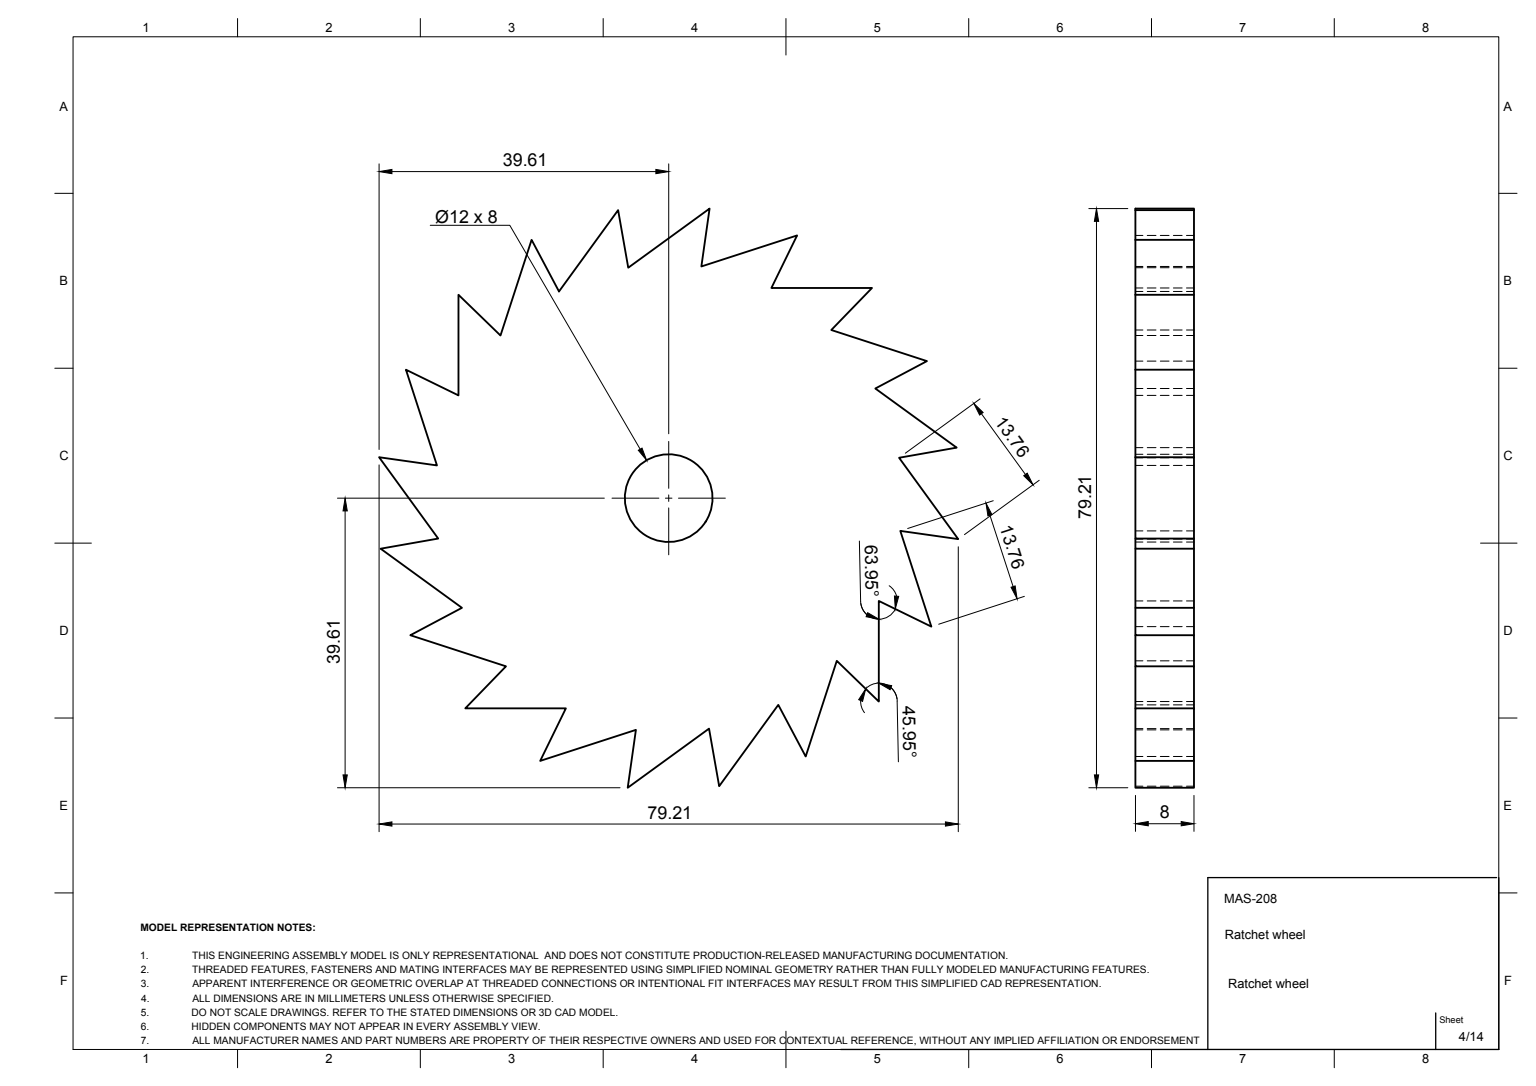
ISO-10303-21;
HEADER;
/* Generated by software containing ST-Developer
 * from STEP Tools, Inc. (www.steptools.com) 
 */

FILE_DESCRIPTION(
/* description */ ('Independent vertical20-tooth ratchet advance with repeated integral-c
ounterweight gravity pawls, swinging drive lever, bronze sleeves and f
ully retained axle stacks.18degpertooth. Native revolutes; geometric c
ycle checking rather than automatic contact/rolling dynamics. Gravity 
closing checked from actual pawl center of mass. Backplate/foot suppor
ts unit. Fits, torque, holding force, wear and life unassigned.'),
/* implementation_level */ '2;1');

FILE_NAME(
/* name */ 'Ratchet wheel.step',
/* time_stamp */ '2026-11-09T06:25:53-08:00',
/* author */ (''),
/* organization */ (''),
/* preprocessor_version */ 'ST-DEVELOPER v20.2',
/* originating_system */ 'Autodesk Translation Framework v15.17.0.0',
/* authorisation */ '');

FILE_SCHEMA (('AUTOMOTIVE_DESIGN { 1 0 10303 214 3 1 1 }'));
ENDSEC;

DATA;
#10=MECHANICAL_DESIGN_GEOMETRIC_PRESENTATION_REPRESENTATION('',(#124),#4643);
#96=SHAPE_REPRESENTATION_RELATIONSHIP('SRR','None',#4701,#110);
#110=ADVANCED_BREP_SHAPE_REPRESENTATION('',(#138),#4630);
#124=STYLED_ITEM('',(#4780),#138);
#138=MANIFOLD_SOLID_BREP('Body1',#2660);
#163=FACE_BOUND('',#523,.T.);
#164=FACE_BOUND('',#525,.T.);
#202=PLANE('',#2862);
#203=PLANE('',#2863);
#204=PLANE('',#2864);
#205=PLANE('',#2865);
#206=PLANE('',#2866);
#207=PLANE('',#2867);
#208=PLANE('',#2868);
#209=PLANE('',#2869);
#210=PLANE('',#2870);
#211=PLANE('',#2871);
#212=PLANE('',#2872);
#213=PLANE('',#2873);
#214=PLANE('',#2874);
#215=PLANE('',#2875);
#216=PLANE('',#2876);
#217=PLANE('',#2877);
#218=PLANE('',#2878);
#219=PLANE('',#2879);
#220=PLANE('',#2880);
#221=PLANE('',#2881);
#222=PLANE('',#2882);
#223=PLANE('',#2883);
#224=PLANE('',#2884);
#225=PLANE('',#2885);
#226=PLANE('',#2886);
#227=PLANE('',#2887);
#228=PLANE('',#2888);
#229=PLANE('',#2889);
#230=PLANE('',#2890);
#231=PLANE('',#2891);
#232=PLANE('',#2892);
#233=PLANE('',#2893);
#234=PLANE('',#2894);
#235=PLANE('',#2895);
#236=PLANE('',#2896);
#237=PLANE('',#2897);
#238=PLANE('',#2898);
#239=PLANE('',#2899);
#240=PLANE('',#2900);
#241=PLANE('',#2901);
#242=PLANE('',#2902);
#243=PLANE('',#2903);
#320=FACE_OUTER_BOUND('',#481,.T.);
#321=FACE_OUTER_BOUND('',#482,.T.);
#322=FACE_OUTER_BOUND('',#483,.T.);
#323=FACE_OUTER_BOUND('',#484,.T.);
#324=FACE_OUTER_BOUND('',#485,.T.);
#325=FACE_OUTER_BOUND('',#486,.T.);
#326=FACE_OUTER_BOUND('',#487,.T.);
#327=FACE_OUTER_BOUND('',#488,.T.);
#328=FACE_OUTER_BOUND('',#489,.T.);
#329=FACE_OUTER_BOUND('',#490,.T.);
#330=FACE_OUTER_BOUND('',#491,.T.);
#331=FACE_OUTER_BOUND('',#492,.T.);
#332=FACE_OUTER_BOUND('',#493,.T.);
#333=FACE_OUTER_BOUND('',#494,.T.);
#334=FACE_OUTER_BOUND('',#495,.T.);
#335=FACE_OUTER_BOUND('',#496,.T.);
#336=FACE_OUTER_BOUND('',#497,.T.);
#337=FACE_OUTER_BOUND('',#498,.T.);
#338=FACE_OUTER_BOUND('',#499,.T.);
#339=FACE_OUTER_BOUND('',#500,.T.);
#340=FACE_OUTER_BOUND('',#501,.T.);
#341=FACE_OUTER_BOUND('',#502,.T.);
#342=FACE_OUTER_BOUND('',#503,.T.);
#343=FACE_OUTER_BOUND('',#504,.T.);
#344=FACE_OUTER_BOUND('',#505,.T.);
#345=FACE_OUTER_BOUND('',#506,.T.);
#346=FACE_OUTER_BOUND('',#507,.T.);
#347=FACE_OUTER_BOUND('',#508,.T.);
#348=FACE_OUTER_BOUND('',#509,.T.);
#349=FACE_OUTER_BOUND('',#510,.T.);
#350=FACE_OUTER_BOUND('',#511,.T.);
#351=FACE_OUTER_BOUND('',#512,.T.);
#352=FACE_OUTER_BOUND('',#513,.T.);
#353=FACE_OUTER_BOUND('',#514,.T.);
#354=FACE_OUTER_BOUND('',#515,.T.);
#355=FACE_OUTER_BOUND('',#516,.T.);
#356=FACE_OUTER_BOUND('',#517,.T.);
#357=FACE_OUTER_BOUND('',#518,.T.);
#358=FACE_OUTER_BOUND('',#519,.T.);
#359=FACE_OUTER_BOUND('',#520,.T.);
#360=FACE_OUTER_BOUND('',#521,.T.);
#361=FACE_OUTER_BOUND('',#522,.T.);
#362=FACE_OUTER_BOUND('',#524,.T.);
#481=EDGE_LOOP('',(#1885,#1886,#1887,#1888));
#482=EDGE_LOOP('',(#1889,#1890,#1891,#1892));
#483=EDGE_LOOP('',(#1893,#1894,#1895,#1896));
#484=EDGE_LOOP('',(#1897,#1898,#1899,#1900));
#485=EDGE_LOOP('',(#1901,#1902,#1903,#1904));
#486=EDGE_LOOP('',(#1905,#1906,#1907,#1908));
#487=EDGE_LOOP('',(#1909,#1910,#1911,#1912));
#488=EDGE_LOOP('',(#1913,#1914,#1915,#1916));
#489=EDGE_LOOP('',(#1917,#1918,#1919,#1920));
#490=EDGE_LOOP('',(#1921,#1922,#1923,#1924));
#491=EDGE_LOOP('',(#1925,#1926,#1927,#1928));
#492=EDGE_LOOP('',(#1929,#1930,#1931,#1932));
#493=EDGE_LOOP('',(#1933,#1934,#1935,#1936));
#494=EDGE_LOOP('',(#1937,#1938,#1939,#1940));
#495=EDGE_LOOP('',(#1941,#1942,#1943,#1944));
#496=EDGE_LOOP('',(#1945,#1946,#1947,#1948));
#497=EDGE_LOOP('',(#1949,#1950,#1951,#1952));
#498=EDGE_LOOP('',(#1953,#1954,#1955,#1956));
#499=EDGE_LOOP('',(#1957,#1958,#1959,#1960));
#500=EDGE_LOOP('',(#1961,#1962,#1963,#1964));
#501=EDGE_LOOP('',(#1965,#1966,#1967,#1968));
#502=EDGE_LOOP('',(#1969,#1970,#1971,#1972));
#503=EDGE_LOOP('',(#1973,#1974,#1975,#1976));
#504=EDGE_LOOP('',(#1977,#1978,#1979,#1980));
#505=EDGE_LOOP('',(#1981,#1982,#1983,#1984));
#506=EDGE_LOOP('',(#1985,#1986,#1987,#1988));
#507=EDGE_LOOP('',(#1989,#1990,#1991,#1992));
#508=EDGE_LOOP('',(#1993,#1994,#1995,#1996));
#509=EDGE_LOOP('',(#1997,#1998,#1999,#2000));
#510=EDGE_LOOP('',(#2001,#2002,#2003,#2004));
#511=EDGE_LOOP('',(#2005,#2006,#2007,#2008));
#512=EDGE_LOOP('',(#2009,#2010,#2011,#2012));
#513=EDGE_LOOP('',(#2013,#2014,#2015,#2016));
#514=EDGE_LOOP('',(#2017,#2018,#2019,#2020));
#515=EDGE_LOOP('',(#2021,#2022,#2023,#2024));
#516=EDGE_LOOP('',(#2025,#2026,#2027,#2028));
#517=EDGE_LOOP('',(#2029,#2030,#2031,#2032));
#518=EDGE_LOOP('',(#2033,#2034,#2035,#2036));
#519=EDGE_LOOP('',(#2037,#2038,#2039,#2040));
#520=EDGE_LOOP('',(#2041,#2042,#2043,#2044));
#521=EDGE_LOOP('',(#2045,#2046,#2047,#2048));
#522=EDGE_LOOP('',(#2049,#2050,#2051,#2052,#2053,#2054,#2055,#2056,#2057,
#2058,#2059,#2060,#2061,#2062,#2063,#2064,#2065,#2066,#2067,#2068,#2069,
#2070,#2071,#2072,#2073,#2074,#2075,#2076,#2077,#2078,#2079,#2080,#2081,
#2082,#2083,#2084,#2085,#2086,#2087,#2088));
#523=EDGE_LOOP('',(#2089));
#524=EDGE_LOOP('',(#2090,#2091,#2092,#2093,#2094,#2095,#2096,#2097,#2098,
#2099,#2100,#2101,#2102,#2103,#2104,#2105,#2106,#2107,#2108,#2109,#2110,
#2111,#2112,#2113,#2114,#2115,#2116,#2117,#2118,#2119,#2120,#2121,#2122,
#2123,#2124,#2125,#2126,#2127,#2128,#2129));
#525=EDGE_LOOP('',(#2130));
#673=LINE('',#3960,#935);
#674=LINE('',#3965,#936);
#675=LINE('',#3967,#937);
#676=LINE('',#3969,#938);
#677=LINE('',#3970,#939);
#678=LINE('',#3973,#940);
#679=LINE('',#3975,#941);
#680=LINE('',#3976,#942);
#681=LINE('',#3979,#943);
#682=LINE('',#3981,#944);
#683=LINE('',#3982,#945);
#684=LINE('',#3985,#946);
#685=LINE('',#3987,#947);
#686=LINE('',#3988,#948);
#687=LINE('',#3991,#949);
#688=LINE('',#3993,#950);
#689=LINE('',#3994,#951);
#690=LINE('',#3997,#952);
#691=LINE('',#3999,#953);
#692=LINE('',#4000,#954);
#693=LINE('',#4003,#955);
#694=LINE('',#4005,#956);
#695=LINE('',#4006,#957);
#696=LINE('',#4009,#958);
#697=LINE('',#4011,#959);
#698=LINE('',#4012,#960);
#699=LINE('',#4015,#961);
#700=LINE('',#4017,#962);
#701=LINE('',#4018,#963);
#702=LINE('',#4021,#964);
#703=LINE('',#4023,#965);
#704=LINE('',#4024,#966);
#705=LINE('',#4027,#967);
#706=LINE('',#4029,#968);
#707=LINE('',#4030,#969);
#708=LINE('',#4033,#970);
#709=LINE('',#4035,#971);
#710=LINE('',#4036,#972);
#711=LINE('',#4039,#973);
#712=LINE('',#4041,#974);
#713=LINE('',#4042,#975);
#714=LINE('',#4045,#976);
#715=LINE('',#4047,#977);
#716=LINE('',#4048,#978);
#717=LINE('',#4051,#979);
#718=LINE('',#4053,#980);
#719=LINE('',#4054,#981);
#720=LINE('',#4057,#982);
#721=LINE('',#4059,#983);
#722=LINE('',#4060,#984);
#723=LINE('',#4063,#985);
#724=LINE('',#4065,#986);
#725=LINE('',#4066,#987);
#726=LINE('',#4069,#988);
#727=LINE('',#4071,#989);
#728=LINE('',#4072,#990);
#729=LINE('',#4075,#991);
#730=LINE('',#4077,#992);
#731=LINE('',#4078,#993);
#732=LINE('',#4081,#994);
#733=LINE('',#4083,#995);
#734=LINE('',#4084,#996);
#735=LINE('',#4087,#997);
#736=LINE('',#4089,#998);
#737=LINE('',#4090,#999);
#738=LINE('',#4093,#1000);
#739=LINE('',#4095,#1001);
#740=LINE('',#4096,#1002);
#741=LINE('',#4099,#1003);
#742=LINE('',#4101,#1004);
#743=LINE('',#4102,#1005);
#744=LINE('',#4105,#1006);
#745=LINE('',#4107,#1007);
#746=LINE('',#4108,#1008);
#747=LINE('',#4111,#1009);
#748=LINE('',#4113,#1010);
#749=LINE('',#4114,#1011);
#750=LINE('',#4117,#1012);
#751=LINE('',#4119,#1013);
#752=LINE('',#4120,#1014);
#753=LINE('',#4123,#1015);
#754=LINE('',#4125,#1016);
#755=LINE('',#4126,#1017);
#756=LINE('',#4129,#1018);
#757=LINE('',#4131,#1019);
#758=LINE('',#4132,#1020);
#759=LINE('',#4135,#1021);
#760=LINE('',#4137,#1022);
#761=LINE('',#4138,#1023);
#762=LINE('',#4141,#1024);
#763=LINE('',#4143,#1025);
#764=LINE('',#4144,#1026);
#765=LINE('',#4147,#1027);
#766=LINE('',#4149,#1028);
#767=LINE('',#4150,#1029);
#768=LINE('',#4153,#1030);
#769=LINE('',#4155,#1031);
#770=LINE('',#4156,#1032);
#771=LINE('',#4159,#1033);
#772=LINE('',#4161,#1034);
#773=LINE('',#4162,#1035);
#774=LINE('',#4165,#1036);
#775=LINE('',#4167,#1037);
#776=LINE('',#4168,#1038);
#777=LINE('',#4171,#1039);
#778=LINE('',#4173,#1040);
#779=LINE('',#4174,#1041);
#780=LINE('',#4177,#1042);
#781=LINE('',#4179,#1043);
#782=LINE('',#4180,#1044);
#783=LINE('',#4183,#1045);
#784=LINE('',#4185,#1046);
#785=LINE('',#4186,#1047);
#786=LINE('',#4189,#1048);
#787=LINE('',#4191,#1049);
#788=LINE('',#4192,#1050);
#789=LINE('',#4195,#1051);
#790=LINE('',#4197,#1052);
#791=LINE('',#4198,#1053);
#792=LINE('',#4200,#1054);
#793=LINE('',#4201,#1055);
#935=VECTOR('',#3183,6.);
#936=VECTOR('',#3188,10.);
#937=VECTOR('',#3189,10.);
#938=VECTOR('',#3190,10.);
#939=VECTOR('',#3191,10.);
#940=VECTOR('',#3194,10.);
#941=VECTOR('',#3195,10.);
#942=VECTOR('',#3196,10.);
#943=VECTOR('',#3199,10.);
#944=VECTOR('',#3200,10.);
#945=VECTOR('',#3201,10.);
#946=VECTOR('',#3204,10.);
#947=VECTOR('',#3205,10.);
#948=VECTOR('',#3206,10.);
#949=VECTOR('',#3209,10.);
#950=VECTOR('',#3210,10.);
#951=VECTOR('',#3211,10.);
#952=VECTOR('',#3214,10.);
#953=VECTOR('',#3215,10.);
#954=VECTOR('',#3216,10.);
#955=VECTOR('',#3219,10.);
#956=VECTOR('',#3220,10.);
#957=VECTOR('',#3221,10.);
#958=VECTOR('',#3224,10.);
#959=VECTOR('',#3225,10.);
#960=VECTOR('',#3226,10.);
#961=VECTOR('',#3229,10.);
#962=VECTOR('',#3230,10.);
#963=VECTOR('',#3231,10.);
#964=VECTOR('',#3234,10.);
#965=VECTOR('',#3235,10.);
#966=VECTOR('',#3236,10.);
#967=VECTOR('',#3239,10.);
#968=VECTOR('',#3240,10.);
#969=VECTOR('',#3241,10.);
#970=VECTOR('',#3244,10.);
#971=VECTOR('',#3245,10.);
#972=VECTOR('',#3246,10.);
#973=VECTOR('',#3249,10.);
#974=VECTOR('',#3250,10.);
#975=VECTOR('',#3251,10.);
#976=VECTOR('',#3254,10.);
#977=VECTOR('',#3255,10.);
#978=VECTOR('',#3256,10.);
#979=VECTOR('',#3259,10.);
#980=VECTOR('',#3260,10.);
#981=VECTOR('',#3261,10.);
#982=VECTOR('',#3264,10.);
#983=VECTOR('',#3265,10.);
#984=VECTOR('',#3266,10.);
#985=VECTOR('',#3269,10.);
#986=VECTOR('',#3270,10.);
#987=VECTOR('',#3271,10.);
#988=VECTOR('',#3274,10.);
#989=VECTOR('',#3275,10.);
#990=VECTOR('',#3276,10.);
#991=VECTOR('',#3279,10.);
#992=VECTOR('',#3280,10.);
#993=VECTOR('',#3281,10.);
#994=VECTOR('',#3284,10.);
#995=VECTOR('',#3285,10.);
#996=VECTOR('',#3286,10.);
#997=VECTOR('',#3289,10.);
#998=VECTOR('',#3290,10.);
#999=VECTOR('',#3291,10.);
#1000=VECTOR('',#3294,10.);
#1001=VECTOR('',#3295,10.);
#1002=VECTOR('',#3296,10.);
#1003=VECTOR('',#3299,10.);
#1004=VECTOR('',#3300,10.);
#1005=VECTOR('',#3301,10.);
#1006=VECTOR('',#3304,10.);
#1007=VECTOR('',#3305,10.);
#1008=VECTOR('',#3306,10.);
#1009=VECTOR('',#3309,10.);
#1010=VECTOR('',#3310,10.);
#1011=VECTOR('',#3311,10.);
#1012=VECTOR('',#3314,10.);
#1013=VECTOR('',#3315,10.);
#1014=VECTOR('',#3316,10.);
#1015=VECTOR('',#3319,10.);
#1016=VECTOR('',#3320,10.);
#1017=VECTOR('',#3321,10.);
#1018=VECTOR('',#3324,10.);
#1019=VECTOR('',#3325,10.);
#1020=VECTOR('',#3326,10.);
#1021=VECTOR('',#3329,10.);
#1022=VECTOR('',#3330,10.);
#1023=VECTOR('',#3331,10.);
#1024=VECTOR('',#3334,10.);
#1025=VECTOR('',#3335,10.);
#1026=VECTOR('',#3336,10.);
#1027=VECTOR('',#3339,10.);
#1028=VECTOR('',#3340,10.);
#1029=VECTOR('',#3341,10.);
#1030=VECTOR('',#3344,10.);
#1031=VECTOR('',#3345,10.);
#1032=VECTOR('',#3346,10.);
#1033=VECTOR('',#3349,10.);
#1034=VECTOR('',#3350,10.);
#1035=VECTOR('',#3351,10.);
#1036=VECTOR('',#3354,10.);
#1037=VECTOR('',#3355,10.);
#1038=VECTOR('',#3356,10.);
#1039=VECTOR('',#3359,10.);
#1040=VECTOR('',#3360,10.);
#1041=VECTOR('',#3361,10.);
#1042=VECTOR('',#3364,10.);
#1043=VECTOR('',#3365,10.);
#1044=VECTOR('',#3366,10.);
#1045=VECTOR('',#3369,10.);
#1046=VECTOR('',#3370,10.);
#1047=VECTOR('',#3371,10.);
#1048=VECTOR('',#3374,10.);
#1049=VECTOR('',#3375,10.);
#1050=VECTOR('',#3376,10.);
#1051=VECTOR('',#3379,10.);
#1052=VECTOR('',#3380,10.);
#1053=VECTOR('',#3381,10.);
#1054=VECTOR('',#3384,10.);
#1055=VECTOR('',#3385,10.);
#1179=CIRCLE('',#2860,6.);
#1180=CIRCLE('',#2861,6.);
#1269=VERTEX_POINT('',#3957);
#1270=VERTEX_POINT('',#3959);
#1271=VERTEX_POINT('',#3963);
#1272=VERTEX_POINT('',#3964);
#1273=VERTEX_POINT('',#3966);
#1274=VERTEX_POINT('',#3968);
#1275=VERTEX_POINT('',#3972);
#1276=VERTEX_POINT('',#3974);
#1277=VERTEX_POINT('',#3978);
#1278=VERTEX_POINT('',#3980);
#1279=VERTEX_POINT('',#3984);
#1280=VERTEX_POINT('',#3986);
#1281=VERTEX_POINT('',#3990);
#1282=VERTEX_POINT('',#3992);
#1283=VERTEX_POINT('',#3996);
#1284=VERTEX_POINT('',#3998);
#1285=VERTEX_POINT('',#4002);
#1286=VERTEX_POINT('',#4004);
#1287=VERTEX_POINT('',#4008);
#1288=VERTEX_POINT('',#4010);
#1289=VERTEX_POINT('',#4014);
#1290=VERTEX_POINT('',#4016);
#1291=VERTEX_POINT('',#4020);
#1292=VERTEX_POINT('',#4022);
#1293=VERTEX_POINT('',#4026);
#1294=VERTEX_POINT('',#4028);
#1295=VERTEX_POINT('',#4032);
#1296=VERTEX_POINT('',#4034);
#1297=VERTEX_POINT('',#4038);
#1298=VERTEX_POINT('',#4040);
#1299=VERTEX_POINT('',#4044);
#1300=VERTEX_POINT('',#4046);
#1301=VERTEX_POINT('',#4050);
#1302=VERTEX_POINT('',#4052);
#1303=VERTEX_POINT('',#4056);
#1304=VERTEX_POINT('',#4058);
#1305=VERTEX_POINT('',#4062);
#1306=VERTEX_POINT('',#4064);
#1307=VERTEX_POINT('',#4068);
#1308=VERTEX_POINT('',#4070);
#1309=VERTEX_POINT('',#4074);
#1310=VERTEX_POINT('',#4076);
#1311=VERTEX_POINT('',#4080);
#1312=VERTEX_POINT('',#4082);
#1313=VERTEX_POINT('',#4086);
#1314=VERTEX_POINT('',#4088);
#1315=VERTEX_POINT('',#4092);
#1316=VERTEX_POINT('',#4094);
#1317=VERTEX_POINT('',#4098);
#1318=VERTEX_POINT('',#4100);
#1319=VERTEX_POINT('',#4104);
#1320=VERTEX_POINT('',#4106);
#1321=VERTEX_POINT('',#4110);
#1322=VERTEX_POINT('',#4112);
#1323=VERTEX_POINT('',#4116);
#1324=VERTEX_POINT('',#4118);
#1325=VERTEX_POINT('',#4122);
#1326=VERTEX_POINT('',#4124);
#1327=VERTEX_POINT('',#4128);
#1328=VERTEX_POINT('',#4130);
#1329=VERTEX_POINT('',#4134);
#1330=VERTEX_POINT('',#4136);
#1331=VERTEX_POINT('',#4140);
#1332=VERTEX_POINT('',#4142);
#1333=VERTEX_POINT('',#4146);
#1334=VERTEX_POINT('',#4148);
#1335=VERTEX_POINT('',#4152);
#1336=VERTEX_POINT('',#4154);
#1337=VERTEX_POINT('',#4158);
#1338=VERTEX_POINT('',#4160);
#1339=VERTEX_POINT('',#4164);
#1340=VERTEX_POINT('',#4166);
#1341=VERTEX_POINT('',#4170);
#1342=VERTEX_POINT('',#4172);
#1343=VERTEX_POINT('',#4176);
#1344=VERTEX_POINT('',#4178);
#1345=VERTEX_POINT('',#4182);
#1346=VERTEX_POINT('',#4184);
#1347=VERTEX_POINT('',#4188);
#1348=VERTEX_POINT('',#4190);
#1349=VERTEX_POINT('',#4194);
#1350=VERTEX_POINT('',#4196);
#1507=EDGE_CURVE('',#1269,#1269,#1179,.T.);
#1508=EDGE_CURVE('',#1269,#1270,#673,.T.);
#1509=EDGE_CURVE('',#1270,#1270,#1180,.T.);
#1510=EDGE_CURVE('',#1271,#1272,#674,.T.);
#1511=EDGE_CURVE('',#1272,#1273,#675,.T.);
#1512=EDGE_CURVE('',#1274,#1273,#676,.T.);
#1513=EDGE_CURVE('',#1271,#1274,#677,.T.);
#1514=EDGE_CURVE('',#1275,#1271,#678,.T.);
#1515=EDGE_CURVE('',#1276,#1274,#679,.T.);
#1516=EDGE_CURVE('',#1275,#1276,#680,.T.);
#1517=EDGE_CURVE('',#1277,#1275,#681,.T.);
#1518=EDGE_CURVE('',#1278,#1276,#682,.T.);
#1519=EDGE_CURVE('',#1277,#1278,#683,.T.);
#1520=EDGE_CURVE('',#1279,#1277,#684,.T.);
#1521=EDGE_CURVE('',#1280,#1278,#685,.T.);
#1522=EDGE_CURVE('',#1279,#1280,#686,.T.);
#1523=EDGE_CURVE('',#1281,#1279,#687,.T.);
#1524=EDGE_CURVE('',#1282,#1280,#688,.T.);
#1525=EDGE_CURVE('',#1281,#1282,#689,.T.);
#1526=EDGE_CURVE('',#1283,#1281,#690,.T.);
#1527=EDGE_CURVE('',#1284,#1282,#691,.T.);
#1528=EDGE_CURVE('',#1283,#1284,#692,.T.);
#1529=EDGE_CURVE('',#1285,#1283,#693,.T.);
#1530=EDGE_CURVE('',#1286,#1284,#694,.T.);
#1531=EDGE_CURVE('',#1285,#1286,#695,.T.);
#1532=EDGE_CURVE('',#1287,#1285,#696,.T.);
#1533=EDGE_CURVE('',#1288,#1286,#697,.T.);
#1534=EDGE_CURVE('',#1287,#1288,#698,.T.);
#1535=EDGE_CURVE('',#1289,#1287,#699,.T.);
#1536=EDGE_CURVE('',#1290,#1288,#700,.T.);
#1537=EDGE_CURVE('',#1289,#1290,#701,.T.);
#1538=EDGE_CURVE('',#1291,#1289,#702,.T.);
#1539=EDGE_CURVE('',#1292,#1290,#703,.T.);
#1540=EDGE_CURVE('',#1291,#1292,#704,.T.);
#1541=EDGE_CURVE('',#1293,#1291,#705,.T.);
#1542=EDGE_CURVE('',#1294,#1292,#706,.T.);
#1543=EDGE_CURVE('',#1293,#1294,#707,.T.);
#1544=EDGE_CURVE('',#1295,#1293,#708,.T.);
#1545=EDGE_CURVE('',#1296,#1294,#709,.T.);
#1546=EDGE_CURVE('',#1295,#1296,#710,.T.);
#1547=EDGE_CURVE('',#1297,#1295,#711,.T.);
#1548=EDGE_CURVE('',#1298,#1296,#712,.T.);
#1549=EDGE_CURVE('',#1297,#1298,#713,.T.);
#1550=EDGE_CURVE('',#1299,#1297,#714,.T.);
#1551=EDGE_CURVE('',#1300,#1298,#715,.T.);
#1552=EDGE_CURVE('',#1299,#1300,#716,.T.);
#1553=EDGE_CURVE('',#1301,#1299,#717,.T.);
#1554=EDGE_CURVE('',#1302,#1300,#718,.T.);
#1555=EDGE_CURVE('',#1301,#1302,#719,.T.);
#1556=EDGE_CURVE('',#1303,#1301,#720,.T.);
#1557=EDGE_CURVE('',#1304,#1302,#721,.T.);
#1558=EDGE_CURVE('',#1303,#1304,#722,.T.);
#1559=EDGE_CURVE('',#1305,#1303,#723,.T.);
#1560=EDGE_CURVE('',#1306,#1304,#724,.T.);
#1561=EDGE_CURVE('',#1305,#1306,#725,.T.);
#1562=EDGE_CURVE('',#1307,#1305,#726,.T.);
#1563=EDGE_CURVE('',#1308,#1306,#727,.T.);
#1564=EDGE_CURVE('',#1307,#1308,#728,.T.);
#1565=EDGE_CURVE('',#1309,#1307,#729,.T.);
#1566=EDGE_CURVE('',#1310,#1308,#730,.T.);
#1567=EDGE_CURVE('',#1309,#1310,#731,.T.);
#1568=EDGE_CURVE('',#1311,#1309,#732,.T.);
#1569=EDGE_CURVE('',#1312,#1310,#733,.T.);
#1570=EDGE_CURVE('',#1311,#1312,#734,.T.);
#1571=EDGE_CURVE('',#1313,#1311,#735,.T.);
#1572=EDGE_CURVE('',#1314,#1312,#736,.T.);
#1573=EDGE_CURVE('',#1313,#1314,#737,.T.);
#1574=EDGE_CURVE('',#1315,#1313,#738,.T.);
#1575=EDGE_CURVE('',#1316,#1314,#739,.T.);
#1576=EDGE_CURVE('',#1315,#1316,#740,.T.);
#1577=EDGE_CURVE('',#1317,#1315,#741,.T.);
#1578=EDGE_CURVE('',#1318,#1316,#742,.T.);
#1579=EDGE_CURVE('',#1317,#1318,#743,.T.);
#1580=EDGE_CURVE('',#1319,#1317,#744,.T.);
#1581=EDGE_CURVE('',#1320,#1318,#745,.T.);
#1582=EDGE_CURVE('',#1319,#1320,#746,.T.);
#1583=EDGE_CURVE('',#1321,#1319,#747,.T.);
#1584=EDGE_CURVE('',#1322,#1320,#748,.T.);
#1585=EDGE_CURVE('',#1321,#1322,#749,.T.);
#1586=EDGE_CURVE('',#1323,#1321,#750,.T.);
#1587=EDGE_CURVE('',#1324,#1322,#751,.T.);
#1588=EDGE_CURVE('',#1323,#1324,#752,.T.);
#1589=EDGE_CURVE('',#1325,#1323,#753,.T.);
#1590=EDGE_CURVE('',#1326,#1324,#754,.T.);
#1591=EDGE_CURVE('',#1325,#1326,#755,.T.);
#1592=EDGE_CURVE('',#1327,#1325,#756,.T.);
#1593=EDGE_CURVE('',#1328,#1326,#757,.T.);
#1594=EDGE_CURVE('',#1327,#1328,#758,.T.);
#1595=EDGE_CURVE('',#1329,#1327,#759,.T.);
#1596=EDGE_CURVE('',#1330,#1328,#760,.T.);
#1597=EDGE_CURVE('',#1329,#1330,#761,.T.);
#1598=EDGE_CURVE('',#1331,#1329,#762,.T.);
#1599=EDGE_CURVE('',#1332,#1330,#763,.T.);
#1600=EDGE_CURVE('',#1331,#1332,#764,.T.);
#1601=EDGE_CURVE('',#1333,#1331,#765,.T.);
#1602=EDGE_CURVE('',#1334,#1332,#766,.T.);
#1603=EDGE_CURVE('',#1333,#1334,#767,.T.);
#1604=EDGE_CURVE('',#1335,#1333,#768,.T.);
#1605=EDGE_CURVE('',#1336,#1334,#769,.T.);
#1606=EDGE_CURVE('',#1335,#1336,#770,.T.);
#1607=EDGE_CURVE('',#1337,#1335,#771,.T.);
#1608=EDGE_CURVE('',#1338,#1336,#772,.T.);
#1609=EDGE_CURVE('',#1337,#1338,#773,.T.);
#1610=EDGE_CURVE('',#1339,#1337,#774,.T.);
#1611=EDGE_CURVE('',#1340,#1338,#775,.T.);
#1612=EDGE_CURVE('',#1339,#1340,#776,.T.);
#1613=EDGE_CURVE('',#1341,#1339,#777,.T.);
#1614=EDGE_CURVE('',#1342,#1340,#778,.T.);
#1615=EDGE_CURVE('',#1341,#1342,#779,.T.);
#1616=EDGE_CURVE('',#1343,#1341,#780,.T.);
#1617=EDGE_CURVE('',#1344,#1342,#781,.T.);
#1618=EDGE_CURVE('',#1343,#1344,#782,.T.);
#1619=EDGE_CURVE('',#1345,#1343,#783,.T.);
#1620=EDGE_CURVE('',#1346,#1344,#784,.T.);
#1621=EDGE_CURVE('',#1345,#1346,#785,.T.);
#1622=EDGE_CURVE('',#1347,#1345,#786,.T.);
#1623=EDGE_CURVE('',#1348,#1346,#787,.T.);
#1624=EDGE_CURVE('',#1347,#1348,#788,.T.);
#1625=EDGE_CURVE('',#1349,#1347,#789,.T.);
#1626=EDGE_CURVE('',#1350,#1348,#790,.T.);
#1627=EDGE_CURVE('',#1349,#1350,#791,.T.);
#1628=EDGE_CURVE('',#1272,#1349,#792,.T.);
#1629=EDGE_CURVE('',#1273,#1350,#793,.T.);
#1885=ORIENTED_EDGE('',*,*,#1507,.F.);
#1886=ORIENTED_EDGE('',*,*,#1508,.T.);
#1887=ORIENTED_EDGE('',*,*,#1509,.F.);
#1888=ORIENTED_EDGE('',*,*,#1508,.F.);
#1889=ORIENTED_EDGE('',*,*,#1510,.T.);
#1890=ORIENTED_EDGE('',*,*,#1511,.T.);
#1891=ORIENTED_EDGE('',*,*,#1512,.F.);
#1892=ORIENTED_EDGE('',*,*,#1513,.F.);
#1893=ORIENTED_EDGE('',*,*,#1514,.T.);
#1894=ORIENTED_EDGE('',*,*,#1513,.T.);
#1895=ORIENTED_EDGE('',*,*,#1515,.F.);
#1896=ORIENTED_EDGE('',*,*,#1516,.F.);
#1897=ORIENTED_EDGE('',*,*,#1517,.T.);
#1898=ORIENTED_EDGE('',*,*,#1516,.T.);
#1899=ORIENTED_EDGE('',*,*,#1518,.F.);
#1900=ORIENTED_EDGE('',*,*,#1519,.F.);
#1901=ORIENTED_EDGE('',*,*,#1520,.T.);
#1902=ORIENTED_EDGE('',*,*,#1519,.T.);
#1903=ORIENTED_EDGE('',*,*,#1521,.F.);
#1904=ORIENTED_EDGE('',*,*,#1522,.F.);
#1905=ORIENTED_EDGE('',*,*,#1523,.T.);
#1906=ORIENTED_EDGE('',*,*,#1522,.T.);
#1907=ORIENTED_EDGE('',*,*,#1524,.F.);
#1908=ORIENTED_EDGE('',*,*,#1525,.F.);
#1909=ORIENTED_EDGE('',*,*,#1526,.T.);
#1910=ORIENTED_EDGE('',*,*,#1525,.T.);
#1911=ORIENTED_EDGE('',*,*,#1527,.F.);
#1912=ORIENTED_EDGE('',*,*,#1528,.F.);
#1913=ORIENTED_EDGE('',*,*,#1529,.T.);
#1914=ORIENTED_EDGE('',*,*,#1528,.T.);
#1915=ORIENTED_EDGE('',*,*,#1530,.F.);
#1916=ORIENTED_EDGE('',*,*,#1531,.F.);
#1917=ORIENTED_EDGE('',*,*,#1532,.T.);
#1918=ORIENTED_EDGE('',*,*,#1531,.T.);
#1919=ORIENTED_EDGE('',*,*,#1533,.F.);
#1920=ORIENTED_EDGE('',*,*,#1534,.F.);
#1921=ORIENTED_EDGE('',*,*,#1535,.T.);
#1922=ORIENTED_EDGE('',*,*,#1534,.T.);
#1923=ORIENTED_EDGE('',*,*,#1536,.F.);
#1924=ORIENTED_EDGE('',*,*,#1537,.F.);
#1925=ORIENTED_EDGE('',*,*,#1538,.T.);
#1926=ORIENTED_EDGE('',*,*,#1537,.T.);
#1927=ORIENTED_EDGE('',*,*,#1539,.F.);
#1928=ORIENTED_EDGE('',*,*,#1540,.F.);
#1929=ORIENTED_EDGE('',*,*,#1541,.T.);
#1930=ORIENTED_EDGE('',*,*,#1540,.T.);
#1931=ORIENTED_EDGE('',*,*,#1542,.F.);
#1932=ORIENTED_EDGE('',*,*,#1543,.F.);
#1933=ORIENTED_EDGE('',*,*,#1544,.T.);
#1934=ORIENTED_EDGE('',*,*,#1543,.T.);
#1935=ORIENTED_EDGE('',*,*,#1545,.F.);
#1936=ORIENTED_EDGE('',*,*,#1546,.F.);
#1937=ORIENTED_EDGE('',*,*,#1547,.T.);
#1938=ORIENTED_EDGE('',*,*,#1546,.T.);
#1939=ORIENTED_EDGE('',*,*,#1548,.F.);
#1940=ORIENTED_EDGE('',*,*,#1549,.F.);
#1941=ORIENTED_EDGE('',*,*,#1550,.T.);
#1942=ORIENTED_EDGE('',*,*,#1549,.T.);
#1943=ORIENTED_EDGE('',*,*,#1551,.F.);
#1944=ORIENTED_EDGE('',*,*,#1552,.F.);
#1945=ORIENTED_EDGE('',*,*,#1553,.T.);
#1946=ORIENTED_EDGE('',*,*,#1552,.T.);
#1947=ORIENTED_EDGE('',*,*,#1554,.F.);
#1948=ORIENTED_EDGE('',*,*,#1555,.F.);
#1949=ORIENTED_EDGE('',*,*,#1556,.T.);
#1950=ORIENTED_EDGE('',*,*,#1555,.T.);
#1951=ORIENTED_EDGE('',*,*,#1557,.F.);
#1952=ORIENTED_EDGE('',*,*,#1558,.F.);
#1953=ORIENTED_EDGE('',*,*,#1559,.T.);
#1954=ORIENTED_EDGE('',*,*,#1558,.T.);
#1955=ORIENTED_EDGE('',*,*,#1560,.F.);
#1956=ORIENTED_EDGE('',*,*,#1561,.F.);
#1957=ORIENTED_EDGE('',*,*,#1562,.T.);
#1958=ORIENTED_EDGE('',*,*,#1561,.T.);
#1959=ORIENTED_EDGE('',*,*,#1563,.F.);
#1960=ORIENTED_EDGE('',*,*,#1564,.F.);
#1961=ORIENTED_EDGE('',*,*,#1565,.T.);
#1962=ORIENTED_EDGE('',*,*,#1564,.T.);
#1963=ORIENTED_EDGE('',*,*,#1566,.F.);
#1964=ORIENTED_EDGE('',*,*,#1567,.F.);
#1965=ORIENTED_EDGE('',*,*,#1568,.T.);
#1966=ORIENTED_EDGE('',*,*,#1567,.T.);
#1967=ORIENTED_EDGE('',*,*,#1569,.F.);
#1968=ORIENTED_EDGE('',*,*,#1570,.F.);
#1969=ORIENTED_EDGE('',*,*,#1571,.T.);
#1970=ORIENTED_EDGE('',*,*,#1570,.T.);
#1971=ORIENTED_EDGE('',*,*,#1572,.F.);
#1972=ORIENTED_EDGE('',*,*,#1573,.F.);
#1973=ORIENTED_EDGE('',*,*,#1574,.T.);
#1974=ORIENTED_EDGE('',*,*,#1573,.T.);
#1975=ORIENTED_EDGE('',*,*,#1575,.F.);
#1976=ORIENTED_EDGE('',*,*,#1576,.F.);
#1977=ORIENTED_EDGE('',*,*,#1577,.T.);
#1978=ORIENTED_EDGE('',*,*,#1576,.T.);
#1979=ORIENTED_EDGE('',*,*,#1578,.F.);
#1980=ORIENTED_EDGE('',*,*,#1579,.F.);
#1981=ORIENTED_EDGE('',*,*,#1580,.T.);
#1982=ORIENTED_EDGE('',*,*,#1579,.T.);
#1983=ORIENTED_EDGE('',*,*,#1581,.F.);
#1984=ORIENTED_EDGE('',*,*,#1582,.F.);
#1985=ORIENTED_EDGE('',*,*,#1583,.T.);
#1986=ORIENTED_EDGE('',*,*,#1582,.T.);
#1987=ORIENTED_EDGE('',*,*,#1584,.F.);
#1988=ORIENTED_EDGE('',*,*,#1585,.F.);
#1989=ORIENTED_EDGE('',*,*,#1586,.T.);
#1990=ORIENTED_EDGE('',*,*,#1585,.T.);
#1991=ORIENTED_EDGE('',*,*,#1587,.F.);
#1992=ORIENTED_EDGE('',*,*,#1588,.F.);
#1993=ORIENTED_EDGE('',*,*,#1589,.T.);
#1994=ORIENTED_EDGE('',*,*,#1588,.T.);
#1995=ORIENTED_EDGE('',*,*,#1590,.F.);
#1996=ORIENTED_EDGE('',*,*,#1591,.F.);
#1997=ORIENTED_EDGE('',*,*,#1592,.T.);
#1998=ORIENTED_EDGE('',*,*,#1591,.T.);
#1999=ORIENTED_EDGE('',*,*,#1593,.F.);
#2000=ORIENTED_EDGE('',*,*,#1594,.F.);
#2001=ORIENTED_EDGE('',*,*,#1595,.T.);
#2002=ORIENTED_EDGE('',*,*,#1594,.T.);
#2003=ORIENTED_EDGE('',*,*,#1596,.F.);
#2004=ORIENTED_EDGE('',*,*,#1597,.F.);
#2005=ORIENTED_EDGE('',*,*,#1598,.T.);
#2006=ORIENTED_EDGE('',*,*,#1597,.T.);
#2007=ORIENTED_EDGE('',*,*,#1599,.F.);
#2008=ORIENTED_EDGE('',*,*,#1600,.F.);
#2009=ORIENTED_EDGE('',*,*,#1601,.T.);
#2010=ORIENTED_EDGE('',*,*,#1600,.T.);
#2011=ORIENTED_EDGE('',*,*,#1602,.F.);
#2012=ORIENTED_EDGE('',*,*,#1603,.F.);
#2013=ORIENTED_EDGE('',*,*,#1604,.T.);
#2014=ORIENTED_EDGE('',*,*,#1603,.T.);
#2015=ORIENTED_EDGE('',*,*,#1605,.F.);
#2016=ORIENTED_EDGE('',*,*,#1606,.F.);
#2017=ORIENTED_EDGE('',*,*,#1607,.T.);
#2018=ORIENTED_EDGE('',*,*,#1606,.T.);
#2019=ORIENTED_EDGE('',*,*,#1608,.F.);
#2020=ORIENTED_EDGE('',*,*,#1609,.F.);
#2021=ORIENTED_EDGE('',*,*,#1610,.T.);
#2022=ORIENTED_EDGE('',*,*,#1609,.T.);
#2023=ORIENTED_EDGE('',*,*,#1611,.F.);
#2024=ORIENTED_EDGE('',*,*,#1612,.F.);
#2025=ORIENTED_EDGE('',*,*,#1613,.T.);
#2026=ORIENTED_EDGE('',*,*,#1612,.T.);
#2027=ORIENTED_EDGE('',*,*,#1614,.F.);
#2028=ORIENTED_EDGE('',*,*,#1615,.F.);
#2029=ORIENTED_EDGE('',*,*,#1616,.T.);
#2030=ORIENTED_EDGE('',*,*,#1615,.T.);
#2031=ORIENTED_EDGE('',*,*,#1617,.F.);
#2032=ORIENTED_EDGE('',*,*,#1618,.F.);
#2033=ORIENTED_EDGE('',*,*,#1619,.T.);
#2034=ORIENTED_EDGE('',*,*,#1618,.T.);
#2035=ORIENTED_EDGE('',*,*,#1620,.F.);
#2036=ORIENTED_EDGE('',*,*,#1621,.F.);
#2037=ORIENTED_EDGE('',*,*,#1622,.T.);
#2038=ORIENTED_EDGE('',*,*,#1621,.T.);
#2039=ORIENTED_EDGE('',*,*,#1623,.F.);
#2040=ORIENTED_EDGE('',*,*,#1624,.F.);
#2041=ORIENTED_EDGE('',*,*,#1625,.T.);
#2042=ORIENTED_EDGE('',*,*,#1624,.T.);
#2043=ORIENTED_EDGE('',*,*,#1626,.F.);
#2044=ORIENTED_EDGE('',*,*,#1627,.F.);
#2045=ORIENTED_EDGE('',*,*,#1628,.T.);
#2046=ORIENTED_EDGE('',*,*,#1627,.T.);
#2047=ORIENTED_EDGE('',*,*,#1629,.F.);
#2048=ORIENTED_EDGE('',*,*,#1511,.F.);
#2049=ORIENTED_EDGE('',*,*,#1629,.T.);
#2050=ORIENTED_EDGE('',*,*,#1626,.T.);
#2051=ORIENTED_EDGE('',*,*,#1623,.T.);
#2052=ORIENTED_EDGE('',*,*,#1620,.T.);
#2053=ORIENTED_EDGE('',*,*,#1617,.T.);
#2054=ORIENTED_EDGE('',*,*,#1614,.T.);
#2055=ORIENTED_EDGE('',*,*,#1611,.T.);
#2056=ORIENTED_EDGE('',*,*,#1608,.T.);
#2057=ORIENTED_EDGE('',*,*,#1605,.T.);
#2058=ORIENTED_EDGE('',*,*,#1602,.T.);
#2059=ORIENTED_EDGE('',*,*,#1599,.T.);
#2060=ORIENTED_EDGE('',*,*,#1596,.T.);
#2061=ORIENTED_EDGE('',*,*,#1593,.T.);
#2062=ORIENTED_EDGE('',*,*,#1590,.T.);
#2063=ORIENTED_EDGE('',*,*,#1587,.T.);
#2064=ORIENTED_EDGE('',*,*,#1584,.T.);
#2065=ORIENTED_EDGE('',*,*,#1581,.T.);
#2066=ORIENTED_EDGE('',*,*,#1578,.T.);
#2067=ORIENTED_EDGE('',*,*,#1575,.T.);
#2068=ORIENTED_EDGE('',*,*,#1572,.T.);
#2069=ORIENTED_EDGE('',*,*,#1569,.T.);
#2070=ORIENTED_EDGE('',*,*,#1566,.T.);
#2071=ORIENTED_EDGE('',*,*,#1563,.T.);
#2072=ORIENTED_EDGE('',*,*,#1560,.T.);
#2073=ORIENTED_EDGE('',*,*,#1557,.T.);
#2074=ORIENTED_EDGE('',*,*,#1554,.T.);
#2075=ORIENTED_EDGE('',*,*,#1551,.T.);
#2076=ORIENTED_EDGE('',*,*,#1548,.T.);
#2077=ORIENTED_EDGE('',*,*,#1545,.T.);
#2078=ORIENTED_EDGE('',*,*,#1542,.T.);
#2079=ORIENTED_EDGE('',*,*,#1539,.T.);
#2080=ORIENTED_EDGE('',*,*,#1536,.T.);
#2081=ORIENTED_EDGE('',*,*,#1533,.T.);
#2082=ORIENTED_EDGE('',*,*,#1530,.T.);
#2083=ORIENTED_EDGE('',*,*,#1527,.T.);
#2084=ORIENTED_EDGE('',*,*,#1524,.T.);
#2085=ORIENTED_EDGE('',*,*,#1521,.T.);
#2086=ORIENTED_EDGE('',*,*,#1518,.T.);
#2087=ORIENTED_EDGE('',*,*,#1515,.T.);
#2088=ORIENTED_EDGE('',*,*,#1512,.T.);
#2089=ORIENTED_EDGE('',*,*,#1507,.T.);
#2090=ORIENTED_EDGE('',*,*,#1628,.F.);
#2091=ORIENTED_EDGE('',*,*,#1510,.F.);
#2092=ORIENTED_EDGE('',*,*,#1514,.F.);
#2093=ORIENTED_EDGE('',*,*,#1517,.F.);
#2094=ORIENTED_EDGE('',*,*,#1520,.F.);
#2095=ORIENTED_EDGE('',*,*,#1523,.F.);
#2096=ORIENTED_EDGE('',*,*,#1526,.F.);
#2097=ORIENTED_EDGE('',*,*,#1529,.F.);
#2098=ORIENTED_EDGE('',*,*,#1532,.F.);
#2099=ORIENTED_EDGE('',*,*,#1535,.F.);
#2100=ORIENTED_EDGE('',*,*,#1538,.F.);
#2101=ORIENTED_EDGE('',*,*,#1541,.F.);
#2102=ORIENTED_EDGE('',*,*,#1544,.F.);
#2103=ORIENTED_EDGE('',*,*,#1547,.F.);
#2104=ORIENTED_EDGE('',*,*,#1550,.F.);
#2105=ORIENTED_EDGE('',*,*,#1553,.F.);
#2106=ORIENTED_EDGE('',*,*,#1556,.F.);
#2107=ORIENTED_EDGE('',*,*,#1559,.F.);
#2108=ORIENTED_EDGE('',*,*,#1562,.F.);
#2109=ORIENTED_EDGE('',*,*,#1565,.F.);
#2110=ORIENTED_EDGE('',*,*,#1568,.F.);
#2111=ORIENTED_EDGE('',*,*,#1571,.F.);
#2112=ORIENTED_EDGE('',*,*,#1574,.F.);
#2113=ORIENTED_EDGE('',*,*,#1577,.F.);
#2114=ORIENTED_EDGE('',*,*,#1580,.F.);
#2115=ORIENTED_EDGE('',*,*,#1583,.F.);
#2116=ORIENTED_EDGE('',*,*,#1586,.F.);
#2117=ORIENTED_EDGE('',*,*,#1589,.F.);
#2118=ORIENTED_EDGE('',*,*,#1592,.F.);
#2119=ORIENTED_EDGE('',*,*,#1595,.F.);
#2120=ORIENTED_EDGE('',*,*,#1598,.F.);
#2121=ORIENTED_EDGE('',*,*,#1601,.F.);
#2122=ORIENTED_EDGE('',*,*,#1604,.F.);
#2123=ORIENTED_EDGE('',*,*,#1607,.F.);
#2124=ORIENTED_EDGE('',*,*,#1610,.F.);
#2125=ORIENTED_EDGE('',*,*,#1613,.F.);
#2126=ORIENTED_EDGE('',*,*,#1616,.F.);
#2127=ORIENTED_EDGE('',*,*,#1619,.F.);
#2128=ORIENTED_EDGE('',*,*,#1622,.F.);
#2129=ORIENTED_EDGE('',*,*,#1625,.F.);
#2130=ORIENTED_EDGE('',*,*,#1509,.T.);
#2479=CYLINDRICAL_SURFACE('',#2859,6.);
#2526=ADVANCED_FACE('',(#320),#2479,.F.);
#2527=ADVANCED_FACE('',(#321),#202,.T.);
#2528=ADVANCED_FACE('',(#322),#203,.T.);
#2529=ADVANCED_FACE('',(#323),#204,.T.);
#2530=ADVANCED_FACE('',(#324),#205,.T.);
#2531=ADVANCED_FACE('',(#325),#206,.T.);
#2532=ADVANCED_FACE('',(#326),#207,.T.);
#2533=ADVANCED_FACE('',(#327),#208,.T.);
#2534=ADVANCED_FACE('',(#328),#209,.T.);
#2535=ADVANCED_FACE('',(#329),#210,.T.);
#2536=ADVANCED_FACE('',(#330),#211,.T.);
#2537=ADVANCED_FACE('',(#331),#212,.T.);
#2538=ADVANCED_FACE('',(#332),#213,.T.);
#2539=ADVANCED_FACE('',(#333),#214,.T.);
#2540=ADVANCED_FACE('',(#334),#215,.T.);
#2541=ADVANCED_FACE('',(#335),#216,.T.);
#2542=ADVANCED_FACE('',(#336),#217,.T.);
#2543=ADVANCED_FACE('',(#337),#218,.T.);
#2544=ADVANCED_FACE('',(#338),#219,.T.);
#2545=ADVANCED_FACE('',(#339),#220,.T.);
#2546=ADVANCED_FACE('',(#340),#221,.T.);
#2547=ADVANCED_FACE('',(#341),#222,.T.);
#2548=ADVANCED_FACE('',(#342),#223,.T.);
#2549=ADVANCED_FACE('',(#343),#224,.T.);
#2550=ADVANCED_FACE('',(#344),#225,.T.);
#2551=ADVANCED_FACE('',(#345),#226,.T.);
#2552=ADVANCED_FACE('',(#346),#227,.T.);
#2553=ADVANCED_FACE('',(#347),#228,.T.);
#2554=ADVANCED_FACE('',(#348),#229,.T.);
#2555=ADVANCED_FACE('',(#349),#230,.T.);
#2556=ADVANCED_FACE('',(#350),#231,.T.);
#2557=ADVANCED_FACE('',(#351),#232,.T.);
#2558=ADVANCED_FACE('',(#352),#233,.T.);
#2559=ADVANCED_FACE('',(#353),#234,.T.);
#2560=ADVANCED_FACE('',(#354),#235,.T.);
#2561=ADVANCED_FACE('',(#355),#236,.T.);
#2562=ADVANCED_FACE('',(#356),#237,.T.);
#2563=ADVANCED_FACE('',(#357),#238,.T.);
#2564=ADVANCED_FACE('',(#358),#239,.T.);
#2565=ADVANCED_FACE('',(#359),#240,.T.);
#2566=ADVANCED_FACE('',(#360),#241,.T.);
#2567=ADVANCED_FACE('',(#361,#163),#242,.T.);
#2568=ADVANCED_FACE('',(#362,#164),#243,.F.);
#2660=CLOSED_SHELL('',(#2526,#2527,#2528,#2529,#2530,#2531,#2532,#2533,
#2534,#2535,#2536,#2537,#2538,#2539,#2540,#2541,#2542,#2543,#2544,#2545,
#2546,#2547,#2548,#2549,#2550,#2551,#2552,#2553,#2554,#2555,#2556,#2557,
#2558,#2559,#2560,#2561,#2562,#2563,#2564,#2565,#2566,#2567,#2568));
#2858=AXIS2_PLACEMENT_3D('',#3955,#3177,#3178);
#2859=AXIS2_PLACEMENT_3D('',#3956,#3179,#3180);
#2860=AXIS2_PLACEMENT_3D('',#3958,#3181,#3182);
#2861=AXIS2_PLACEMENT_3D('',#3961,#3184,#3185);
#2862=AXIS2_PLACEMENT_3D('',#3962,#3186,#3187);
#2863=AXIS2_PLACEMENT_3D('',#3971,#3192,#3193);
#2864=AXIS2_PLACEMENT_3D('',#3977,#3197,#3198);
#2865=AXIS2_PLACEMENT_3D('',#3983,#3202,#3203);
#2866=AXIS2_PLACEMENT_3D('',#3989,#3207,#3208);
#2867=AXIS2_PLACEMENT_3D('',#3995,#3212,#3213);
#2868=AXIS2_PLACEMENT_3D('',#4001,#3217,#3218);
#2869=AXIS2_PLACEMENT_3D('',#4007,#3222,#3223);
#2870=AXIS2_PLACEMENT_3D('',#4013,#3227,#3228);
#2871=AXIS2_PLACEMENT_3D('',#4019,#3232,#3233);
#2872=AXIS2_PLACEMENT_3D('',#4025,#3237,#3238);
#2873=AXIS2_PLACEMENT_3D('',#4031,#3242,#3243);
#2874=AXIS2_PLACEMENT_3D('',#4037,#3247,#3248);
#2875=AXIS2_PLACEMENT_3D('',#4043,#3252,#3253);
#2876=AXIS2_PLACEMENT_3D('',#4049,#3257,#3258);
#2877=AXIS2_PLACEMENT_3D('',#4055,#3262,#3263);
#2878=AXIS2_PLACEMENT_3D('',#4061,#3267,#3268);
#2879=AXIS2_PLACEMENT_3D('',#4067,#3272,#3273);
#2880=AXIS2_PLACEMENT_3D('',#4073,#3277,#3278);
#2881=AXIS2_PLACEMENT_3D('',#4079,#3282,#3283);
#2882=AXIS2_PLACEMENT_3D('',#4085,#3287,#3288);
#2883=AXIS2_PLACEMENT_3D('',#4091,#3292,#3293);
#2884=AXIS2_PLACEMENT_3D('',#4097,#3297,#3298);
#2885=AXIS2_PLACEMENT_3D('',#4103,#3302,#3303);
#2886=AXIS2_PLACEMENT_3D('',#4109,#3307,#3308);
#2887=AXIS2_PLACEMENT_3D('',#4115,#3312,#3313);
#2888=AXIS2_PLACEMENT_3D('',#4121,#3317,#3318);
#2889=AXIS2_PLACEMENT_3D('',#4127,#3322,#3323);
#2890=AXIS2_PLACEMENT_3D('',#4133,#3327,#3328);
#2891=AXIS2_PLACEMENT_3D('',#4139,#3332,#3333);
#2892=AXIS2_PLACEMENT_3D('',#4145,#3337,#3338);
#2893=AXIS2_PLACEMENT_3D('',#4151,#3342,#3343);
#2894=AXIS2_PLACEMENT_3D('',#4157,#3347,#3348);
#2895=AXIS2_PLACEMENT_3D('',#4163,#3352,#3353);
#2896=AXIS2_PLACEMENT_3D('',#4169,#3357,#3358);
#2897=AXIS2_PLACEMENT_3D('',#4175,#3362,#3363);
#2898=AXIS2_PLACEMENT_3D('',#4181,#3367,#3368);
#2899=AXIS2_PLACEMENT_3D('',#4187,#3372,#3373);
#2900=AXIS2_PLACEMENT_3D('',#4193,#3377,#3378);
#2901=AXIS2_PLACEMENT_3D('',#4199,#3382,#3383);
#2902=AXIS2_PLACEMENT_3D('',#4202,#3386,#3387);
#2903=AXIS2_PLACEMENT_3D('',#4203,#3388,#3389);
#3177=DIRECTION('axis',(0.,0.,1.));
#3178=DIRECTION('refdir',(1.,0.,0.));
#3179=DIRECTION('center_axis',(0.,0.,-1.));
#3180=DIRECTION('ref_axis',(1.,0.,0.));
#3181=DIRECTION('center_axis',(0.,0.,-1.));
#3182=DIRECTION('ref_axis',(1.,0.,0.));
#3183=DIRECTION('',(0.,0.,-1.));
#3184=DIRECTION('center_axis',(0.,0.,1.));
#3185=DIRECTION('ref_axis',(1.,0.,0.));
#3186=DIRECTION('center_axis',(-0.309016994374948,-0.951056516295153,0.));
#3187=DIRECTION('ref_axis',(0.951056516295153,-0.309016994374948,0.));
#3188=DIRECTION('',(0.951056516295153,-0.309016994374948,0.));
#3189=DIRECTION('',(0.,0.,1.));
#3190=DIRECTION('',(0.951056516295153,-0.309016994374948,0.));
#3191=DIRECTION('',(0.,0.,1.));
#3192=DIRECTION('center_axis',(0.990144448700884,0.140049886493426,0.));
#3193=DIRECTION('ref_axis',(-0.140049886493426,0.990144448700885,0.));
#3194=DIRECTION('',(-0.140049886493426,0.990144448700885,0.));
#3195=DIRECTION('',(-0.140049886493426,0.990144448700885,0.));
#3196=DIRECTION('',(0.,0.,1.));
#3197=DIRECTION('center_axis',(-0.587785252292474,-0.809016994374947,0.));
#3198=DIRECTION('ref_axis',(0.809016994374947,-0.587785252292473,0.));
#3199=DIRECTION('',(0.809016994374947,-0.587785252292473,0.));
#3200=DIRECTION('',(0.809016994374947,-0.587785252292473,0.));
#3201=DIRECTION('',(0.,0.,1.));
#3202=DIRECTION('center_axis',(0.9849611249972,-0.172776104378617,0.));
#3203=DIRECTION('ref_axis',(0.172776104378617,0.9849611249972,0.));
#3204=DIRECTION('',(0.172776104378617,0.9849611249972,0.));
#3205=DIRECTION('',(0.172776104378617,0.9849611249972,0.));
#3206=DIRECTION('',(0.,0.,1.));
#3207=DIRECTION('center_axis',(-0.809016994374948,-0.587785252292473,0.));
#3208=DIRECTION('ref_axis',(0.587785252292473,-0.809016994374948,0.));
#3209=DIRECTION('',(0.587785252292473,-0.809016994374948,0.));
#3210=DIRECTION('',(0.587785252292473,-0.809016994374948,0.));
#3211=DIRECTION('',(0.,0.,1.));
#3212=DIRECTION('center_axis',(0.8833629437511,-0.468689566352177,0.));
#3213=DIRECTION('ref_axis',(0.468689566352177,0.8833629437511,0.));
#3214=DIRECTION('',(0.468689566352177,0.8833629437511,0.));
#3215=DIRECTION('',(0.468689566352177,0.8833629437511,0.));
#3216=DIRECTION('',(0.,0.,1.));
#3217=DIRECTION('center_axis',(-0.951056516295154,-0.309016994374947,0.));
#3218=DIRECTION('ref_axis',(0.309016994374947,-0.951056516295154,0.));
#3219=DIRECTION('',(0.309016994374947,-0.951056516295154,0.));
#3220=DIRECTION('',(0.309016994374947,-0.951056516295154,0.));
#3221=DIRECTION('',(0.,0.,1.));
#3222=DIRECTION('center_axis',(0.695295042819105,-0.718724428018958,0.));
#3223=DIRECTION('ref_axis',(0.718724428018958,0.695295042819105,0.));
#3224=DIRECTION('',(0.718724428018958,0.695295042819105,0.));
#3225=DIRECTION('',(0.718724428018958,0.695295042819105,0.));
#3226=DIRECTION('',(0.,0.,1.));
#3227=DIRECTION('center_axis',(-1.,1.83697019872103E-16,0.));
#3228=DIRECTION('ref_axis',(-1.83697019872103E-16,-1.,0.));
#3229=DIRECTION('',(-1.83697019872103E-16,-1.,0.));
#3230=DIRECTION('',(-1.83697019872103E-16,-1.,0.));
#3231=DIRECTION('',(0.,0.,1.));
#3232=DIRECTION('center_axis',(0.439166818690556,-0.898405535023698,0.));
#3233=DIRECTION('ref_axis',(0.898405535023697,0.439166818690556,0.));
#3234=DIRECTION('',(0.898405535023697,0.439166818690556,0.));
#3235=DIRECTION('',(0.898405535023697,0.439166818690556,0.));
#3236=DIRECTION('',(0.,0.,1.));
#3237=DIRECTION('center_axis',(-0.951056516295154,0.309016994374948,0.));
#3238=DIRECTION('ref_axis',(-0.309016994374948,-0.951056516295153,0.));
#3239=DIRECTION('',(-0.309016994374948,-0.951056516295153,0.));
#3240=DIRECTION('',(-0.309016994374948,-0.951056516295153,0.));
#3241=DIRECTION('',(0.,0.,1.));
#3242=DIRECTION('center_axis',(0.140049886493426,-0.990144448700884,0.));
#3243=DIRECTION('ref_axis',(0.990144448700885,0.140049886493426,0.));
#3244=DIRECTION('',(0.990144448700885,0.140049886493426,0.));
#3245=DIRECTION('',(0.990144448700885,0.140049886493426,0.));
#3246=DIRECTION('',(0.,0.,1.));
#3247=DIRECTION('center_axis',(-0.809016994374947,0.587785252292473,0.));
#3248=DIRECTION('ref_axis',(-0.587785252292473,-0.809016994374947,0.));
#3249=DIRECTION('',(-0.587785252292473,-0.809016994374947,0.));
#3250=DIRECTION('',(-0.587785252292473,-0.809016994374947,0.));
#3251=DIRECTION('',(0.,0.,1.));
#3252=DIRECTION('center_axis',(-0.172776104378617,-0.9849611249972,0.));
#3253=DIRECTION('ref_axis',(0.9849611249972,-0.172776104378617,0.));
#3254=DIRECTION('',(0.9849611249972,-0.172776104378617,0.));
#3255=DIRECTION('',(0.9849611249972,-0.172776104378617,0.));
#3256=DIRECTION('',(0.,0.,1.));
#3257=DIRECTION('center_axis',(-0.587785252292473,0.809016994374948,0.));
#3258=DIRECTION('ref_axis',(-0.809016994374947,-0.587785252292473,0.));
#3259=DIRECTION('',(-0.809016994374947,-0.587785252292473,0.));
#3260=DIRECTION('',(-0.809016994374947,-0.587785252292473,0.));
#3261=DIRECTION('',(0.,0.,1.));
#3262=DIRECTION('center_axis',(-0.468689566352177,-0.8833629437511,0.));
#3263=DIRECTION('ref_axis',(0.8833629437511,-0.468689566352176,0.));
#3264=DIRECTION('',(0.8833629437511,-0.468689566352176,0.));
#3265=DIRECTION('',(0.8833629437511,-0.468689566352176,0.));
#3266=DIRECTION('',(0.,0.,1.));
#3267=DIRECTION('center_axis',(-0.309016994374947,0.951056516295154,0.));
#3268=DIRECTION('ref_axis',(-0.951056516295154,-0.309016994374947,0.));
#3269=DIRECTION('',(-0.951056516295154,-0.309016994374947,0.));
#3270=DIRECTION('',(-0.951056516295154,-0.309016994374947,0.));
#3271=DIRECTION('',(0.,0.,1.));
#3272=DIRECTION('center_axis',(-0.718724428018958,-0.695295042819105,0.));
#3273=DIRECTION('ref_axis',(0.695295042819105,-0.718724428018958,0.));
#3274=DIRECTION('',(0.695295042819105,-0.718724428018958,0.));
#3275=DIRECTION('',(0.695295042819105,-0.718724428018958,0.));
#3276=DIRECTION('',(0.,0.,1.));
#3277=DIRECTION('center_axis',(1.22464679914735E-16,1.,0.));
#3278=DIRECTION('ref_axis',(-1.,1.22464679914735E-16,0.));
#3279=DIRECTION('',(-1.,1.22464679914735E-16,0.));
#3280=DIRECTION('',(-1.,1.22464679914735E-16,0.));
#3281=DIRECTION('',(0.,0.,1.));
#3282=DIRECTION('center_axis',(-0.898405535023698,-0.439166818690556,0.));
#3283=DIRECTION('ref_axis',(0.439166818690556,-0.898405535023697,0.));
#3284=DIRECTION('',(0.439166818690556,-0.898405535023697,0.));
#3285=DIRECTION('',(0.439166818690556,-0.898405535023697,0.));
#3286=DIRECTION('',(0.,0.,1.));
#3287=DIRECTION('center_axis',(0.309016994374948,0.951056516295154,0.));
#3288=DIRECTION('ref_axis',(-0.951056516295153,0.309016994374948,0.));
#3289=DIRECTION('',(-0.951056516295153,0.309016994374948,0.));
#3290=DIRECTION('',(-0.951056516295153,0.309016994374948,0.));
#3291=DIRECTION('',(0.,0.,1.));
#3292=DIRECTION('center_axis',(-0.990144448700884,-0.140049886493426,0.));
#3293=DIRECTION('ref_axis',(0.140049886493426,-0.990144448700885,0.));
#3294=DIRECTION('',(0.140049886493426,-0.990144448700885,0.));
#3295=DIRECTION('',(0.140049886493426,-0.990144448700885,0.));
#3296=DIRECTION('',(0.,0.,1.));
#3297=DIRECTION('center_axis',(0.587785252292473,0.809016994374947,0.));
#3298=DIRECTION('ref_axis',(-0.809016994374947,0.587785252292473,0.));
#3299=DIRECTION('',(-0.809016994374947,0.587785252292473,0.));
#3300=DIRECTION('',(-0.809016994374947,0.587785252292473,0.));
#3301=DIRECTION('',(0.,0.,1.));
#3302=DIRECTION('center_axis',(-0.9849611249972,0.172776104378617,0.));
#3303=DIRECTION('ref_axis',(-0.172776104378617,-0.9849611249972,0.));
#3304=DIRECTION('',(-0.172776104378617,-0.9849611249972,0.));
#3305=DIRECTION('',(-0.172776104378617,-0.9849611249972,0.));
#3306=DIRECTION('',(0.,0.,1.));
#3307=DIRECTION('center_axis',(0.809016994374948,0.587785252292473,0.));
#3308=DIRECTION('ref_axis',(-0.587785252292473,0.809016994374947,0.));
#3309=DIRECTION('',(-0.587785252292473,0.809016994374947,0.));
#3310=DIRECTION('',(-0.587785252292473,0.809016994374947,0.));
#3311=DIRECTION('',(0.,0.,1.));
#3312=DIRECTION('center_axis',(-0.8833629437511,0.468689566352176,0.));
#3313=DIRECTION('ref_axis',(-0.468689566352176,-0.8833629437511,0.));
#3314=DIRECTION('',(-0.468689566352176,-0.8833629437511,0.));
#3315=DIRECTION('',(-0.468689566352176,-0.8833629437511,0.));
#3316=DIRECTION('',(0.,0.,1.));
#3317=DIRECTION('center_axis',(0.951056516295154,0.309016994374947,0.));
#3318=DIRECTION('ref_axis',(-0.309016994374947,0.951056516295154,0.));
#3319=DIRECTION('',(-0.309016994374947,0.951056516295154,0.));
#3320=DIRECTION('',(-0.309016994374947,0.951056516295154,0.));
#3321=DIRECTION('',(0.,0.,1.));
#3322=DIRECTION('center_axis',(-0.695295042819106,0.718724428018958,0.));
#3323=DIRECTION('ref_axis',(-0.718724428018958,-0.695295042819106,0.));
#3324=DIRECTION('',(-0.718724428018958,-0.695295042819105,0.));
#3325=DIRECTION('',(-0.718724428018958,-0.695295042819105,0.));
#3326=DIRECTION('',(0.,0.,1.));
#3327=DIRECTION('center_axis',(1.,-6.12323399573677E-17,0.));
#3328=DIRECTION('ref_axis',(6.12323399573677E-17,1.,0.));
#3329=DIRECTION('',(6.12323399573677E-17,1.,0.));
#3330=DIRECTION('',(6.12323399573677E-17,1.,0.));
#3331=DIRECTION('',(0.,0.,1.));
#3332=DIRECTION('center_axis',(-0.439166818690556,0.898405535023698,0.));
#3333=DIRECTION('ref_axis',(-0.898405535023697,-0.439166818690556,0.));
#3334=DIRECTION('',(-0.898405535023697,-0.439166818690556,0.));
#3335=DIRECTION('',(-0.898405535023697,-0.439166818690556,0.));
#3336=DIRECTION('',(0.,0.,1.));
#3337=DIRECTION('center_axis',(0.951056516295154,-0.309016994374948,0.));
#3338=DIRECTION('ref_axis',(0.309016994374948,0.951056516295153,0.));
#3339=DIRECTION('',(0.309016994374948,0.951056516295153,0.));
#3340=DIRECTION('',(0.309016994374948,0.951056516295153,0.));
#3341=DIRECTION('',(0.,0.,1.));
#3342=DIRECTION('center_axis',(-0.140049886493427,0.990144448700884,0.));
#3343=DIRECTION('ref_axis',(-0.990144448700884,-0.140049886493427,0.));
#3344=DIRECTION('',(-0.990144448700884,-0.140049886493427,0.));
#3345=DIRECTION('',(-0.990144448700884,-0.140049886493427,0.));
#3346=DIRECTION('',(0.,0.,1.));
#3347=DIRECTION('center_axis',(0.809016994374948,-0.587785252292473,0.));
#3348=DIRECTION('ref_axis',(0.587785252292473,0.809016994374947,0.));
#3349=DIRECTION('',(0.587785252292473,0.809016994374947,0.));
#3350=DIRECTION('',(0.587785252292473,0.809016994374947,0.));
#3351=DIRECTION('',(0.,0.,1.));
#3352=DIRECTION('center_axis',(0.172776104378617,0.9849611249972,0.));
#3353=DIRECTION('ref_axis',(-0.9849611249972,0.172776104378617,0.));
#3354=DIRECTION('',(-0.9849611249972,0.172776104378617,0.));
#3355=DIRECTION('',(-0.9849611249972,0.172776104378617,0.));
#3356=DIRECTION('',(0.,0.,1.));
#3357=DIRECTION('center_axis',(0.587785252292473,-0.809016994374948,0.));
#3358=DIRECTION('ref_axis',(0.809016994374947,0.587785252292473,0.));
#3359=DIRECTION('',(0.809016994374947,0.587785252292473,0.));
#3360=DIRECTION('',(0.809016994374947,0.587785252292473,0.));
#3361=DIRECTION('',(0.,0.,1.));
#3362=DIRECTION('center_axis',(0.468689566352177,0.8833629437511,0.));
#3363=DIRECTION('ref_axis',(-0.8833629437511,0.468689566352177,0.));
#3364=DIRECTION('',(-0.8833629437511,0.468689566352177,0.));
#3365=DIRECTION('',(-0.8833629437511,0.468689566352177,0.));
#3366=DIRECTION('',(0.,0.,1.));
#3367=DIRECTION('center_axis',(0.309016994374948,-0.951056516295154,0.));
#3368=DIRECTION('ref_axis',(0.951056516295153,0.309016994374948,0.));
#3369=DIRECTION('',(0.951056516295153,0.309016994374948,0.));
#3370=DIRECTION('',(0.951056516295153,0.309016994374948,0.));
#3371=DIRECTION('',(0.,0.,1.));
#3372=DIRECTION('center_axis',(0.718724428018958,0.695295042819106,0.));
#3373=DIRECTION('ref_axis',(-0.695295042819106,0.718724428018958,0.));
#3374=DIRECTION('',(-0.695295042819106,0.718724428018958,0.));
#3375=DIRECTION('',(-0.695295042819106,0.718724428018958,0.));
#3376=DIRECTION('',(0.,0.,1.));
#3377=DIRECTION('center_axis',(0.,-1.,0.));
#3378=DIRECTION('ref_axis',(1.,0.,0.));
#3379=DIRECTION('',(1.,0.,0.));
#3380=DIRECTION('',(1.,0.,0.));
#3381=DIRECTION('',(0.,0.,1.));
#3382=DIRECTION('center_axis',(0.898405535023698,0.439166818690556,0.));
#3383=DIRECTION('ref_axis',(-0.439166818690556,0.898405535023698,0.));
#3384=DIRECTION('',(-0.439166818690556,0.898405535023698,0.));
#3385=DIRECTION('',(-0.439166818690556,0.898405535023698,0.));
#3386=DIRECTION('center_axis',(0.,0.,1.));
#3387=DIRECTION('ref_axis',(1.,0.,0.));
#3388=DIRECTION('center_axis',(0.,0.,1.));
#3389=DIRECTION('ref_axis',(1.,0.,0.));
#3955=CARTESIAN_POINT('',(0.,0.,0.));
#3956=CARTESIAN_POINT('Origin',(0.,0.,4.));
#3957=CARTESIAN_POINT('',(-6.,7.34788079488412E-16,8.));
#3958=CARTESIAN_POINT('Origin',(0.,0.,8.));
#3959=CARTESIAN_POINT('',(-6.,7.34788079488412E-16,0.));
#3960=CARTESIAN_POINT('',(-6.,7.34788079488412E-16,4.));
#3961=CARTESIAN_POINT('Origin',(0.,0.,0.));
#3962=CARTESIAN_POINT('Origin',(30.4338085214449,-9.88854381999833,0.));
#3963=CARTESIAN_POINT('',(30.4338085214449,-9.88854381999833,0.));
#3964=CARTESIAN_POINT('',(38.0422606518061,-12.3606797749979,0.));
#3965=CARTESIAN_POINT('',(30.4338085214449,-9.88854381999833,0.));
#3966=CARTESIAN_POINT('',(38.0422606518061,-12.3606797749979,8.));
#3967=CARTESIAN_POINT('',(38.0422606518061,-12.3606797749979,0.));
#3968=CARTESIAN_POINT('',(30.4338085214449,-9.88854381999833,8.));
#3969=CARTESIAN_POINT('',(30.4338085214449,-9.88854381999833,8.));
#3970=CARTESIAN_POINT('',(30.4338085214449,-9.88854381999833,0.));
#3971=CARTESIAN_POINT('Origin',(32.3606797749979,-23.5114100916989,0.));
#3972=CARTESIAN_POINT('',(32.3606797749979,-23.5114100916989,0.));
#3973=CARTESIAN_POINT('',(32.3606797749979,-23.5114100916989,0.));
#3974=CARTESIAN_POINT('',(32.3606797749979,-23.5114100916989,8.));
#3975=CARTESIAN_POINT('',(32.3606797749979,-23.5114100916989,8.));
#3976=CARTESIAN_POINT('',(32.3606797749979,-23.5114100916989,0.));
#3977=CARTESIAN_POINT('Origin',(25.8885438199983,-18.8091280733591,0.));
#3978=CARTESIAN_POINT('',(25.8885438199983,-18.8091280733591,0.));
#3979=CARTESIAN_POINT('',(25.8885438199983,-18.8091280733591,0.));
#3980=CARTESIAN_POINT('',(25.8885438199983,-18.8091280733591,8.));
#3981=CARTESIAN_POINT('',(25.8885438199983,-18.8091280733591,8.));
#3982=CARTESIAN_POINT('',(25.8885438199983,-18.8091280733591,0.));
#3983=CARTESIAN_POINT('Origin',(23.5114100916989,-32.3606797749979,0.));
#3984=CARTESIAN_POINT('',(23.5114100916989,-32.3606797749979,0.));
#3985=CARTESIAN_POINT('',(23.5114100916989,-32.3606797749979,0.));
#3986=CARTESIAN_POINT('',(23.5114100916989,-32.3606797749979,8.));
#3987=CARTESIAN_POINT('',(23.5114100916989,-32.3606797749979,8.));
#3988=CARTESIAN_POINT('',(23.5114100916989,-32.3606797749979,0.));
#3989=CARTESIAN_POINT('Origin',(18.8091280733591,-25.8885438199983,0.));
#3990=CARTESIAN_POINT('',(18.8091280733591,-25.8885438199983,0.));
#3991=CARTESIAN_POINT('',(18.8091280733591,-25.8885438199983,0.));
#3992=CARTESIAN_POINT('',(18.8091280733591,-25.8885438199983,8.));
#3993=CARTESIAN_POINT('',(18.8091280733591,-25.8885438199983,8.));
#3994=CARTESIAN_POINT('',(18.8091280733591,-25.8885438199983,0.));
#3995=CARTESIAN_POINT('Origin',(12.3606797749979,-38.0422606518061,0.));
#3996=CARTESIAN_POINT('',(12.3606797749979,-38.0422606518061,0.));
#3997=CARTESIAN_POINT('',(12.3606797749979,-38.0422606518061,0.));
#3998=CARTESIAN_POINT('',(12.3606797749979,-38.0422606518061,8.));
#3999=CARTESIAN_POINT('',(12.3606797749979,-38.0422606518061,8.));
#4000=CARTESIAN_POINT('',(12.3606797749979,-38.0422606518061,0.));
#4001=CARTESIAN_POINT('Origin',(9.88854381999831,-30.4338085214449,0.));
#4002=CARTESIAN_POINT('',(9.88854381999831,-30.4338085214449,0.));
#4003=CARTESIAN_POINT('',(9.88854381999831,-30.4338085214449,0.));
#4004=CARTESIAN_POINT('',(9.88854381999831,-30.4338085214449,8.));
#4005=CARTESIAN_POINT('',(9.88854381999831,-30.4338085214449,8.));
#4006=CARTESIAN_POINT('',(9.88854381999831,-30.4338085214449,0.));
#4007=CARTESIAN_POINT('Origin',(-7.34788079488412E-15,-40.,0.));
#4008=CARTESIAN_POINT('',(-7.34788079488412E-15,-40.,0.));
#4009=CARTESIAN_POINT('',(-7.34788079488412E-15,-40.,0.));
#4010=CARTESIAN_POINT('',(-8.88178419700125E-15,-40.,8.));
#4011=CARTESIAN_POINT('',(-7.34788079488412E-15,-40.,8.));
#4012=CARTESIAN_POINT('',(-7.34788079488412E-15,-40.,0.));
#4013=CARTESIAN_POINT('Origin',(-5.8783046359073E-15,-32.,0.));
#4014=CARTESIAN_POINT('',(-5.8783046359073E-15,-32.,0.));
#4015=CARTESIAN_POINT('',(-5.8783046359073E-15,-32.,0.));
#4016=CARTESIAN_POINT('',(-4.44089209850063E-15,-32.,8.));
#4017=CARTESIAN_POINT('',(-5.8783046359073E-15,-32.,8.));
#4018=CARTESIAN_POINT('',(-5.8783046359073E-15,-32.,0.));
#4019=CARTESIAN_POINT('Origin',(-12.3606797749979,-38.0422606518061,0.));
#4020=CARTESIAN_POINT('',(-12.3606797749979,-38.0422606518061,0.));
#4021=CARTESIAN_POINT('',(-12.3606797749979,-38.0422606518061,0.));
#4022=CARTESIAN_POINT('',(-12.3606797749979,-38.0422606518061,8.));
#4023=CARTESIAN_POINT('',(-12.3606797749979,-38.0422606518061,8.));
#4024=CARTESIAN_POINT('',(-12.3606797749979,-38.0422606518061,0.));
#4025=CARTESIAN_POINT('Origin',(-9.88854381999832,-30.4338085214449,0.));
#4026=CARTESIAN_POINT('',(-9.88854381999832,-30.4338085214449,0.));
#4027=CARTESIAN_POINT('',(-9.88854381999832,-30.4338085214449,0.));
#4028=CARTESIAN_POINT('',(-9.88854381999833,-30.4338085214449,8.));
#4029=CARTESIAN_POINT('',(-9.88854381999832,-30.4338085214449,8.));
#4030=CARTESIAN_POINT('',(-9.88854381999832,-30.4338085214449,0.));
#4031=CARTESIAN_POINT('Origin',(-23.5114100916989,-32.3606797749979,0.));
#4032=CARTESIAN_POINT('',(-23.5114100916989,-32.3606797749979,0.));
#4033=CARTESIAN_POINT('',(-23.5114100916989,-32.3606797749979,0.));
#4034=CARTESIAN_POINT('',(-23.5114100916989,-32.3606797749979,8.));
#4035=CARTESIAN_POINT('',(-23.5114100916989,-32.3606797749979,8.));
#4036=CARTESIAN_POINT('',(-23.5114100916989,-32.3606797749979,0.));
#4037=CARTESIAN_POINT('Origin',(-18.8091280733591,-25.8885438199983,0.));
#4038=CARTESIAN_POINT('',(-18.8091280733591,-25.8885438199983,0.));
#4039=CARTESIAN_POINT('',(-18.8091280733591,-25.8885438199983,0.));
#4040=CARTESIAN_POINT('',(-18.8091280733591,-25.8885438199983,8.));
#4041=CARTESIAN_POINT('',(-18.8091280733591,-25.8885438199983,8.));
#4042=CARTESIAN_POINT('',(-18.8091280733591,-25.8885438199983,0.));
#4043=CARTESIAN_POINT('Origin',(-32.3606797749979,-23.5114100916989,0.));
#4044=CARTESIAN_POINT('',(-32.3606797749979,-23.5114100916989,0.));
#4045=CARTESIAN_POINT('',(-32.3606797749979,-23.5114100916989,0.));
#4046=CARTESIAN_POINT('',(-32.3606797749979,-23.5114100916989,8.));
#4047=CARTESIAN_POINT('',(-32.3606797749979,-23.5114100916989,8.));
#4048=CARTESIAN_POINT('',(-32.3606797749979,-23.5114100916989,0.));
#4049=CARTESIAN_POINT('Origin',(-25.8885438199983,-18.8091280733591,0.));
#4050=CARTESIAN_POINT('',(-25.8885438199983,-18.8091280733591,0.));
#4051=CARTESIAN_POINT('',(-25.8885438199983,-18.8091280733591,0.));
#4052=CARTESIAN_POINT('',(-25.8885438199983,-18.8091280733591,8.));
#4053=CARTESIAN_POINT('',(-25.8885438199983,-18.8091280733591,8.));
#4054=CARTESIAN_POINT('',(-25.8885438199983,-18.8091280733591,0.));
#4055=CARTESIAN_POINT('Origin',(-38.0422606518061,-12.3606797749979,0.));
#4056=CARTESIAN_POINT('',(-38.0422606518061,-12.3606797749979,0.));
#4057=CARTESIAN_POINT('',(-38.0422606518061,-12.3606797749979,0.));
#4058=CARTESIAN_POINT('',(-38.0422606518061,-12.3606797749979,8.));
#4059=CARTESIAN_POINT('',(-38.0422606518061,-12.3606797749979,8.));
#4060=CARTESIAN_POINT('',(-38.0422606518061,-12.3606797749979,0.));
#4061=CARTESIAN_POINT('Origin',(-30.4338085214449,-9.88854381999831,0.));
#4062=CARTESIAN_POINT('',(-30.4338085214449,-9.88854381999831,0.));
#4063=CARTESIAN_POINT('',(-30.4338085214449,-9.88854381999831,0.));
#4064=CARTESIAN_POINT('',(-30.4338085214449,-9.88854381999831,8.));
#4065=CARTESIAN_POINT('',(-30.4338085214449,-9.88854381999831,8.));
#4066=CARTESIAN_POINT('',(-30.4338085214449,-9.88854381999831,0.));
#4067=CARTESIAN_POINT('Origin',(-40.,4.89858719658941E-15,0.));
#4068=CARTESIAN_POINT('',(-40.,4.89858719658941E-15,0.));
#4069=CARTESIAN_POINT('',(-40.,4.89858719658941E-15,0.));
#4070=CARTESIAN_POINT('',(-40.,4.44089209850063E-15,8.));
#4071=CARTESIAN_POINT('',(-40.,4.89858719658941E-15,8.));
#4072=CARTESIAN_POINT('',(-40.,4.89858719658941E-15,0.));
#4073=CARTESIAN_POINT('Origin',(-32.,3.91886975727153E-15,0.));
#4074=CARTESIAN_POINT('',(-32.,3.91886975727153E-15,0.));
#4075=CARTESIAN_POINT('',(-32.,3.91886975727153E-15,0.));
#4076=CARTESIAN_POINT('',(-32.,4.44089209850063E-15,8.));
#4077=CARTESIAN_POINT('',(-32.,3.91886975727153E-15,8.));
#4078=CARTESIAN_POINT('',(-32.,3.91886975727153E-15,0.));
#4079=CARTESIAN_POINT('Origin',(-38.0422606518061,12.3606797749979,0.));
#4080=CARTESIAN_POINT('',(-38.0422606518061,12.3606797749979,0.));
#4081=CARTESIAN_POINT('',(-38.0422606518061,12.3606797749979,0.));
#4082=CARTESIAN_POINT('',(-38.0422606518061,12.3606797749979,8.));
#4083=CARTESIAN_POINT('',(-38.0422606518061,12.3606797749979,8.));
#4084=CARTESIAN_POINT('',(-38.0422606518061,12.3606797749979,0.));
#4085=CARTESIAN_POINT('Origin',(-30.4338085214449,9.88854381999832,0.));
#4086=CARTESIAN_POINT('',(-30.4338085214449,9.88854381999832,0.));
#4087=CARTESIAN_POINT('',(-30.4338085214449,9.88854381999832,0.));
#4088=CARTESIAN_POINT('',(-30.4338085214449,9.88854381999832,8.));
#4089=CARTESIAN_POINT('',(-30.4338085214449,9.88854381999832,8.));
#4090=CARTESIAN_POINT('',(-30.4338085214449,9.88854381999832,0.));
#4091=CARTESIAN_POINT('Origin',(-32.3606797749979,23.5114100916989,0.));
#4092=CARTESIAN_POINT('',(-32.3606797749979,23.5114100916989,0.));
#4093=CARTESIAN_POINT('',(-32.3606797749979,23.5114100916989,0.));
#4094=CARTESIAN_POINT('',(-32.3606797749979,23.5114100916989,8.));
#4095=CARTESIAN_POINT('',(-32.3606797749979,23.5114100916989,8.));
#4096=CARTESIAN_POINT('',(-32.3606797749979,23.5114100916989,0.));
#4097=CARTESIAN_POINT('Origin',(-25.8885438199983,18.8091280733591,0.));
#4098=CARTESIAN_POINT('',(-25.8885438199983,18.8091280733591,0.));
#4099=CARTESIAN_POINT('',(-25.8885438199983,18.8091280733591,0.));
#4100=CARTESIAN_POINT('',(-25.8885438199983,18.8091280733591,8.));
#4101=CARTESIAN_POINT('',(-25.8885438199983,18.8091280733591,8.));
#4102=CARTESIAN_POINT('',(-25.8885438199983,18.8091280733591,0.));
#4103=CARTESIAN_POINT('Origin',(-23.5114100916989,32.3606797749979,0.));
#4104=CARTESIAN_POINT('',(-23.5114100916989,32.3606797749979,0.));
#4105=CARTESIAN_POINT('',(-23.5114100916989,32.3606797749979,0.));
#4106=CARTESIAN_POINT('',(-23.5114100916989,32.3606797749979,8.));
#4107=CARTESIAN_POINT('',(-23.5114100916989,32.3606797749979,8.));
#4108=CARTESIAN_POINT('',(-23.5114100916989,32.3606797749979,0.));
#4109=CARTESIAN_POINT('Origin',(-18.8091280733591,25.8885438199983,0.));
#4110=CARTESIAN_POINT('',(-18.8091280733591,25.8885438199983,0.));
#4111=CARTESIAN_POINT('',(-18.8091280733591,25.8885438199983,0.));
#4112=CARTESIAN_POINT('',(-18.8091280733591,25.8885438199983,8.));
#4113=CARTESIAN_POINT('',(-18.8091280733591,25.8885438199983,8.));
#4114=CARTESIAN_POINT('',(-18.8091280733591,25.8885438199983,0.));
#4115=CARTESIAN_POINT('Origin',(-12.3606797749979,38.0422606518061,0.));
#4116=CARTESIAN_POINT('',(-12.3606797749979,38.0422606518061,0.));
#4117=CARTESIAN_POINT('',(-12.3606797749979,38.0422606518061,0.));
#4118=CARTESIAN_POINT('',(-12.3606797749979,38.0422606518061,8.));
#4119=CARTESIAN_POINT('',(-12.3606797749979,38.0422606518061,8.));
#4120=CARTESIAN_POINT('',(-12.3606797749979,38.0422606518061,0.));
#4121=CARTESIAN_POINT('Origin',(-9.88854381999831,30.4338085214449,0.));
#4122=CARTESIAN_POINT('',(-9.88854381999831,30.4338085214449,0.));
#4123=CARTESIAN_POINT('',(-9.88854381999831,30.4338085214449,0.));
#4124=CARTESIAN_POINT('',(-9.88854381999832,30.4338085214449,8.));
#4125=CARTESIAN_POINT('',(-9.88854381999831,30.4338085214449,8.));
#4126=CARTESIAN_POINT('',(-9.88854381999831,30.4338085214449,0.));
#4127=CARTESIAN_POINT('Origin',(2.44929359829471E-15,40.,0.));
#4128=CARTESIAN_POINT('',(2.44929359829471E-15,40.,0.));
#4129=CARTESIAN_POINT('',(2.44929359829471E-15,40.,0.));
#4130=CARTESIAN_POINT('',(4.44089209850063E-15,40.,8.));
#4131=CARTESIAN_POINT('',(2.44929359829471E-15,40.,8.));
#4132=CARTESIAN_POINT('',(2.44929359829471E-15,40.,0.));
#4133=CARTESIAN_POINT('Origin',(1.95943487863577E-15,32.,0.));
#4134=CARTESIAN_POINT('',(1.95943487863577E-15,32.,0.));
#4135=CARTESIAN_POINT('',(1.95943487863577E-15,32.,0.));
#4136=CARTESIAN_POINT('',(0.,32.,8.));
#4137=CARTESIAN_POINT('',(1.95943487863577E-15,32.,8.));
#4138=CARTESIAN_POINT('',(1.95943487863577E-15,32.,0.));
#4139=CARTESIAN_POINT('Origin',(12.3606797749979,38.0422606518061,0.));
#4140=CARTESIAN_POINT('',(12.3606797749979,38.0422606518061,0.));
#4141=CARTESIAN_POINT('',(12.3606797749979,38.0422606518061,0.));
#4142=CARTESIAN_POINT('',(12.3606797749979,38.0422606518061,8.));
#4143=CARTESIAN_POINT('',(12.3606797749979,38.0422606518061,8.));
#4144=CARTESIAN_POINT('',(12.3606797749979,38.0422606518061,0.));
#4145=CARTESIAN_POINT('Origin',(9.88854381999832,30.4338085214449,0.));
#4146=CARTESIAN_POINT('',(9.88854381999832,30.4338085214449,0.));
#4147=CARTESIAN_POINT('',(9.88854381999832,30.4338085214449,0.));
#4148=CARTESIAN_POINT('',(9.88854381999832,30.4338085214449,8.));
#4149=CARTESIAN_POINT('',(9.88854381999832,30.4338085214449,8.));
#4150=CARTESIAN_POINT('',(9.88854381999832,30.4338085214449,0.));
#4151=CARTESIAN_POINT('Origin',(23.5114100916989,32.3606797749979,0.));
#4152=CARTESIAN_POINT('',(23.5114100916989,32.3606797749979,0.));
#4153=CARTESIAN_POINT('',(23.5114100916989,32.3606797749979,0.));
#4154=CARTESIAN_POINT('',(23.5114100916989,32.3606797749979,8.));
#4155=CARTESIAN_POINT('',(23.5114100916989,32.3606797749979,8.));
#4156=CARTESIAN_POINT('',(23.5114100916989,32.3606797749979,0.));
#4157=CARTESIAN_POINT('Origin',(18.8091280733591,25.8885438199983,0.));
#4158=CARTESIAN_POINT('',(18.8091280733591,25.8885438199983,0.));
#4159=CARTESIAN_POINT('',(18.8091280733591,25.8885438199983,0.));
#4160=CARTESIAN_POINT('',(18.8091280733591,25.8885438199983,8.));
#4161=CARTESIAN_POINT('',(18.8091280733591,25.8885438199983,8.));
#4162=CARTESIAN_POINT('',(18.8091280733591,25.8885438199983,0.));
#4163=CARTESIAN_POINT('Origin',(32.3606797749979,23.5114100916989,0.));
#4164=CARTESIAN_POINT('',(32.3606797749979,23.5114100916989,0.));
#4165=CARTESIAN_POINT('',(32.3606797749979,23.5114100916989,0.));
#4166=CARTESIAN_POINT('',(32.3606797749979,23.5114100916989,8.));
#4167=CARTESIAN_POINT('',(32.3606797749979,23.5114100916989,8.));
#4168=CARTESIAN_POINT('',(32.3606797749979,23.5114100916989,0.));
#4169=CARTESIAN_POINT('Origin',(25.8885438199983,18.8091280733591,0.));
#4170=CARTESIAN_POINT('',(25.8885438199983,18.8091280733591,0.));
#4171=CARTESIAN_POINT('',(25.8885438199983,18.8091280733591,0.));
#4172=CARTESIAN_POINT('',(25.8885438199983,18.8091280733591,8.));
#4173=CARTESIAN_POINT('',(25.8885438199983,18.8091280733591,8.));
#4174=CARTESIAN_POINT('',(25.8885438199983,18.8091280733591,0.));
#4175=CARTESIAN_POINT('Origin',(38.0422606518061,12.3606797749979,0.));
#4176=CARTESIAN_POINT('',(38.0422606518061,12.3606797749979,0.));
#4177=CARTESIAN_POINT('',(38.0422606518061,12.3606797749979,0.));
#4178=CARTESIAN_POINT('',(38.0422606518061,12.3606797749979,8.));
#4179=CARTESIAN_POINT('',(38.0422606518061,12.3606797749979,8.));
#4180=CARTESIAN_POINT('',(38.0422606518061,12.3606797749979,0.));
#4181=CARTESIAN_POINT('Origin',(30.4338085214449,9.88854381999832,0.));
#4182=CARTESIAN_POINT('',(30.4338085214449,9.88854381999832,0.));
#4183=CARTESIAN_POINT('',(30.4338085214449,9.88854381999832,0.));
#4184=CARTESIAN_POINT('',(30.4338085214449,9.88854381999832,8.));
#4185=CARTESIAN_POINT('',(30.4338085214449,9.88854381999832,8.));
#4186=CARTESIAN_POINT('',(30.4338085214449,9.88854381999832,0.));
#4187=CARTESIAN_POINT('Origin',(40.,0.,0.));
#4188=CARTESIAN_POINT('',(40.,0.,0.));
#4189=CARTESIAN_POINT('',(40.,0.,0.));
#4190=CARTESIAN_POINT('',(40.,0.,8.));
#4191=CARTESIAN_POINT('',(40.,0.,8.));
#4192=CARTESIAN_POINT('',(40.,0.,0.));
#4193=CARTESIAN_POINT('Origin',(32.,0.,0.));
#4194=CARTESIAN_POINT('',(32.,0.,0.));
#4195=CARTESIAN_POINT('',(32.,0.,0.));
#4196=CARTESIAN_POINT('',(32.,0.,8.));
#4197=CARTESIAN_POINT('',(32.,0.,8.));
#4198=CARTESIAN_POINT('',(32.,0.,0.));
#4199=CARTESIAN_POINT('Origin',(38.0422606518061,-12.3606797749979,0.));
#4200=CARTESIAN_POINT('',(38.0422606518061,-12.3606797749979,0.));
#4201=CARTESIAN_POINT('',(38.0422606518061,-12.3606797749979,8.));
#4202=CARTESIAN_POINT('Origin',(0.,0.,8.));
#4203=CARTESIAN_POINT('Origin',(0.,0.,0.));
#4614=UNCERTAINTY_MEASURE_WITH_UNIT(LENGTH_MEASURE(0.01),#4644,
'DISTANCE_ACCURACY_VALUE',
'Maximum model space distance between geometric entities at asserted c
onnectivities');
#4627=UNCERTAINTY_MEASURE_WITH_UNIT(LENGTH_MEASURE(0.01),#4644,
'DISTANCE_ACCURACY_VALUE',
'Maximum model space distance between geometric entities at asserted c
onnectivities');
#4630=(
GEOMETRIC_REPRESENTATION_CONTEXT(3)
GLOBAL_UNCERTAINTY_ASSIGNED_CONTEXT((#4614))
GLOBAL_UNIT_ASSIGNED_CONTEXT((#4644,#4646,#4647))
REPRESENTATION_CONTEXT('','3D')
);
#4643=(
GEOMETRIC_REPRESENTATION_CONTEXT(3)
GLOBAL_UNCERTAINTY_ASSIGNED_CONTEXT((#4627))
GLOBAL_UNIT_ASSIGNED_CONTEXT((#4644,#4646,#4647))
REPRESENTATION_CONTEXT('','3D')
);
#4644=(
LENGTH_UNIT()
NAMED_UNIT(*)
SI_UNIT(.MILLI.,.METRE.)
);
#4646=(
NAMED_UNIT(*)
PLANE_ANGLE_UNIT()
SI_UNIT($,.RADIAN.)
);
#4647=(
NAMED_UNIT(*)
SI_UNIT($,.STERADIAN.)
SOLID_ANGLE_UNIT()
);
#4650=SHAPE_DEFINITION_REPRESENTATION(#4665,#4701);
#4665=PRODUCT_DEFINITION_SHAPE('',$,#4717);
#4701=SHAPE_REPRESENTATION('',(#2858),#4630);
#4714=PRODUCT_DEFINITION_CONTEXT('part definition',#4761,'design');
#4717=PRODUCT_DEFINITION('Ratchet wheel','Ratchet wheel',#4732,#4714);
#4732=PRODUCT_DEFINITION_FORMATION('',$,#4765);
#4761=APPLICATION_CONTEXT(
'Core Data for Automotive Mechanical Design Process');
#4762=PRODUCT_CONTEXT('part definition',#4761,'mechanical');
#4765=PRODUCT('Ratchet wheel','Ratchet wheel','Ratchet wheel',(#4762));
#4780=PRESENTATION_STYLE_ASSIGNMENT((#4789));
#4789=SURFACE_STYLE_USAGE(.BOTH.,#4798);
#4798=SURFACE_SIDE_STYLE('',(#4807));
#4807=SURFACE_STYLE_FILL_AREA(#4816);
#4816=FILL_AREA_STYLE('Dark blue',(#4825));
#4825=FILL_AREA_STYLE_COLOUR('Dark blue',#4834);
#4834=COLOUR_RGB('Dark blue',0.0901960784313725,0.270588235294118,0.513725490196078);
ENDSEC;
END-ISO-10303-21;
